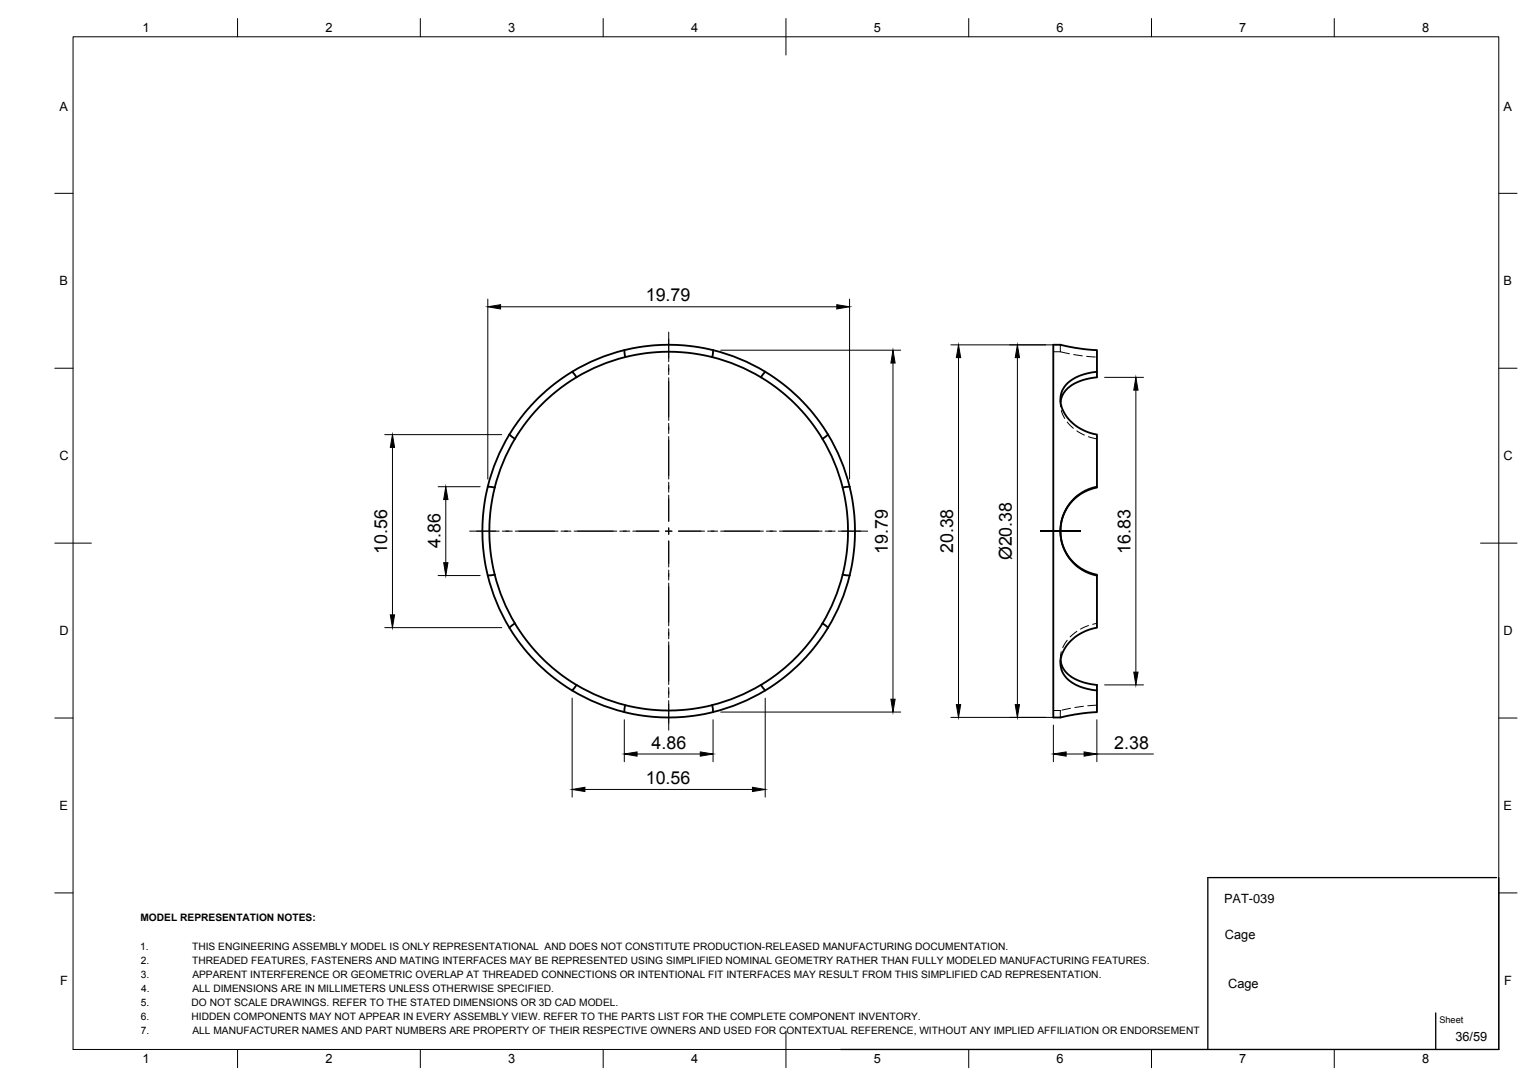
ISO-10303-21;
HEADER;
/* Generated by software containing ST-Developer
 * from STEP Tools, Inc. (www.steptools.com) 
 */

FILE_DESCRIPTION(
/* description */ ('Four-bar parallelogram arm'),
/* implementation_level */ '2;1');

FILE_NAME(
/* name */ 'Cage.step',
/* time_stamp */ '2026-10-28T03:24:55-07:00',
/* author */ (''),
/* organization */ (''),
/* preprocessor_version */ 'ST-DEVELOPER v20.2',
/* originating_system */ 'Autodesk Translation Framework v15.17.0.0',
/* authorisation */ '');

FILE_SCHEMA (('AUTOMOTIVE_DESIGN { 1 0 10303 214 3 1 1 }'));
ENDSEC;

DATA;
#10=MECHANICAL_DESIGN_GEOMETRIC_PRESENTATION_REPRESENTATION('',(#664),#14512);
#467=SPHERICAL_SURFACE('',#8565,0.247676);
#468=SPHERICAL_SURFACE('',#8581,0.247676);
#469=SPHERICAL_SURFACE('',#8586,0.247676);
#470=SPHERICAL_SURFACE('',#8591,0.247676);
#471=SPHERICAL_SURFACE('',#8596,0.247676);
#472=SPHERICAL_SURFACE('',#8601,0.247676);
#473=SPHERICAL_SURFACE('',#8606,0.247676);
#474=SPHERICAL_SURFACE('',#8614,0.247676);
#504=B_SPLINE_CURVE_WITH_KNOTS('',3,(#13344,#13345,#13346,#13347,#13348,
#13349,#13350,#13351,#13352,#13353,#13354,#13355,#13356,#13357,#13358,#13359,
#13360,#13361,#13362,#13363,#13364,#13365),.UNSPECIFIED.,.F.,.F.,(4,2,2,
2,2,2,2,2,2,2,4),(0.0473477652366656,0.126350602536658,0.189525903804987,
0.252701205073317,0.313298422430275,0.373895639787233,0.434492857144191,
0.495090074501149,0.558265375769478,0.621440677037807,0.7004435143378),
 .UNSPECIFIED.);
#505=B_SPLINE_CURVE_WITH_KNOTS('',3,(#13369,#13370,#13371,#13372,#13373,
#13374,#13375,#13376,#13377,#13378,#13379,#13380,#13381,#13382,#13383,#13384,
#13385,#13386,#13387,#13388,#13389,#13390),.UNSPECIFIED.,.F.,.F.,(4,2,2,
2,2,2,2,2,2,2,4),(0.0464897534940957,0.0852567806515119,0.170513561303024,
0.246687263103517,0.308657850341199,0.370628437578881,0.432599024816563,
0.494569612054245,0.570743313854739,0.656000094506251,0.694767121663666),
 .UNSPECIFIED.);
#506=B_SPLINE_CURVE_WITH_KNOTS('',3,(#13396,#13397,#13398,#13399,#13400,
#13401,#13402,#13403,#13404,#13405,#13406,#13407,#13408,#13409,#13410,#13411,
#13412,#13413,#13414,#13415,#13416,#13417),.UNSPECIFIED.,.F.,.F.,(4,2,2,
2,2,2,2,2,2,2,4),(0.0464897534940957,0.0852567806515118,0.170513561303024,
0.246687263103517,0.308657850341199,0.370628437578881,0.432599024816563,
0.494569612054245,0.570743313854738,0.65600009450625,0.694767121663666),
 .UNSPECIFIED.);
#507=B_SPLINE_CURVE_WITH_KNOTS('',3,(#13421,#13422,#13423,#13424,#13425,
#13426,#13427,#13428,#13429,#13430,#13431,#13432,#13433,#13434,#13435,#13436,
#13437,#13438,#13439,#13440,#13441,#13442),.UNSPECIFIED.,.F.,.F.,(4,2,2,
2,2,2,2,2,2,2,4),(0.0464897534940957,0.0852567806515119,0.170513561303024,
0.246687263103517,0.308657850341199,0.370628437578881,0.432599024816563,
0.494569612054245,0.570743313854739,0.656000094506251,0.694767121663666),
 .UNSPECIFIED.);
#508=B_SPLINE_CURVE_WITH_KNOTS('',3,(#13446,#13447,#13448,#13449,#13450,
#13451,#13452,#13453,#13454,#13455,#13456,#13457),.UNSPECIFIED.,.F.,.F.,
(4,2,2,2,2,4),(0.0464897534940957,0.0852567806515119,0.170513561303024,
0.246687263103517,0.308657850341199,0.370628437578881),.UNSPECIFIED.);
#509=B_SPLINE_CURVE_WITH_KNOTS('',3,(#13462,#13463,#13464,#13465,#13466,
#13467,#13468,#13469,#13470,#13471,#13472,#13473),.UNSPECIFIED.,.F.,.F.,
(4,2,2,2,2,4),(0.370628437578881,0.432599024816563,0.494569612054245,0.570743313854738,
0.65600009450625,0.694767121663666),.UNSPECIFIED.);
#510=B_SPLINE_CURVE_WITH_KNOTS('',3,(#13477,#13478,#13479,#13480,#13481,
#13482,#13483,#13484,#13485,#13486,#13487,#13488,#13489,#13490,#13491,#13492,
#13493,#13494,#13495,#13496,#13497,#13498),.UNSPECIFIED.,.F.,.F.,(4,2,2,
2,2,2,2,2,2,2,4),(0.0464897534940957,0.0852567806515121,0.170513561303024,
0.246687263103518,0.308657850341199,0.370628437578881,0.432599024816563,
0.494569612054245,0.570743313854738,0.65600009450625,0.694767121663666),
 .UNSPECIFIED.);
#511=B_SPLINE_CURVE_WITH_KNOTS('',3,(#13502,#13503,#13504,#13505,#13506,
#13507,#13508,#13509,#13510,#13511,#13512,#13513,#13514,#13515,#13516,#13517,
#13518,#13519,#13520,#13521,#13522,#13523),.UNSPECIFIED.,.F.,.F.,(4,2,2,
2,2,2,2,2,2,2,4),(0.0464897534940957,0.0852567806515119,0.170513561303024,
0.246687263103517,0.308657850341199,0.370628437578881,0.432599024816563,
0.494569612054245,0.570743313854738,0.65600009450625,0.694767121663667),
 .UNSPECIFIED.);
#512=B_SPLINE_CURVE_WITH_KNOTS('',3,(#13527,#13528,#13529,#13530,#13531,
#13532,#13533,#13534,#13535,#13536,#13537,#13538,#13539,#13540,#13541,#13542,
#13543,#13544,#13545,#13546,#13547,#13548),.UNSPECIFIED.,.F.,.F.,(4,2,2,
2,2,2,2,2,2,2,4),(0.0464897534940957,0.0852567806515119,0.170513561303024,
0.246687263103517,0.308657850341199,0.370628437578881,0.432599024816563,
0.494569612054245,0.570743313854738,0.65600009450625,0.694767121663666),
 .UNSPECIFIED.);
#513=B_SPLINE_CURVE_WITH_KNOTS('',3,(#13552,#13553,#13554,#13555,#13556,
#13557,#13558,#13559,#13560,#13561,#13562,#13563,#13564,#13565,#13566,#13567,
#13568,#13569,#13570,#13571,#13572,#13573),.UNSPECIFIED.,.F.,.F.,(4,2,2,
2,2,2,2,2,2,2,4),(0.0464897534940957,0.0852567806515119,0.170513561303024,
0.246687263103517,0.308657850341199,0.370628437578881,0.432599024816563,
0.494569612054245,0.570743313854739,0.656000094506251,0.694767121663667),
 .UNSPECIFIED.);
#514=B_SPLINE_CURVE_WITH_KNOTS('',3,(#13581,#13582,#13583,#13584,#13585,
#13586,#13587,#13588,#13589,#13590,#13591,#13592,#13593,#13594,#13595,#13596,
#13597,#13598,#13599,#13600,#13601,#13602),.UNSPECIFIED.,.F.,.F.,(4,2,2,
2,2,2,2,2,2,2,4),(0.0473477652366656,0.126350602536658,0.189525903804987,
0.252701205073316,0.313298422430274,0.373895639787232,0.434492857144191,
0.495090074501149,0.558265375769478,0.621440677037807,0.7004435143378),
 .UNSPECIFIED.);
#515=B_SPLINE_CURVE_WITH_KNOTS('',3,(#13610,#13611,#13612,#13613,#13614,
#13615,#13616,#13617,#13618,#13619,#13620,#13621,#13622,#13623,#13624,#13625,
#13626,#13627,#13628,#13629,#13630,#13631),.UNSPECIFIED.,.F.,.F.,(4,2,2,
2,2,2,2,2,2,2,4),(0.0473477652366656,0.126350602536658,0.189525903804987,
0.252701205073317,0.313298422430275,0.373895639787233,0.434492857144191,
0.495090074501149,0.558265375769478,0.621440677037807,0.7004435143378),
 .UNSPECIFIED.);
#516=B_SPLINE_CURVE_WITH_KNOTS('',3,(#13640,#13641,#13642,#13643,#13644,
#13645,#13646,#13647,#13648,#13649,#13650,#13651),.UNSPECIFIED.,.F.,.F.,
(4,2,2,2,2,4),(0.0473477652366656,0.126350602536658,0.189525903804987,0.252701205073316,
0.313298422430275,0.373895639787233),.UNSPECIFIED.);
#517=B_SPLINE_CURVE_WITH_KNOTS('',3,(#13653,#13654,#13655,#13656,#13657,
#13658,#13659,#13660,#13661,#13662,#13663,#13664),.UNSPECIFIED.,.F.,.F.,
(4,2,2,2,2,4),(0.373895639787233,0.434492857144191,0.495090074501149,0.558265375769478,
0.621440677037807,0.7004435143378),.UNSPECIFIED.);
#518=B_SPLINE_CURVE_WITH_KNOTS('',3,(#13671,#13672,#13673,#13674,#13675,
#13676,#13677,#13678,#13679,#13680,#13681,#13682,#13683,#13684,#13685,#13686,
#13687,#13688,#13689,#13690,#13691,#13692),.UNSPECIFIED.,.F.,.F.,(4,2,2,
2,2,2,2,2,2,2,4),(0.0473477652366656,0.126350602536658,0.189525903804987,
0.252701205073316,0.313298422430275,0.373895639787233,0.434492857144191,
0.495090074501149,0.558265375769478,0.621440677037807,0.7004435143378),
 .UNSPECIFIED.);
#519=B_SPLINE_CURVE_WITH_KNOTS('',3,(#13700,#13701,#13702,#13703,#13704,
#13705,#13706,#13707,#13708,#13709,#13710,#13711,#13712,#13713,#13714,#13715,
#13716,#13717,#13718,#13719,#13720,#13721),.UNSPECIFIED.,.F.,.F.,(4,2,2,
2,2,2,2,2,2,2,4),(0.0473477652366656,0.126350602536658,0.189525903804987,
0.252701205073317,0.313298422430275,0.373895639787233,0.434492857144191,
0.495090074501149,0.558265375769478,0.621440677037807,0.7004435143378),
 .UNSPECIFIED.);
#520=B_SPLINE_CURVE_WITH_KNOTS('',3,(#13729,#13730,#13731,#13732,#13733,
#13734,#13735,#13736,#13737,#13738,#13739,#13740,#13741,#13742,#13743,#13744,
#13745,#13746,#13747,#13748,#13749,#13750),.UNSPECIFIED.,.F.,.F.,(4,2,2,
2,2,2,2,2,2,2,4),(0.0473477652366656,0.126350602536658,0.189525903804987,
0.252701205073316,0.313298422430275,0.373895639787233,0.434492857144191,
0.495090074501149,0.558265375769478,0.621440677037807,0.7004435143378),
 .UNSPECIFIED.);
#521=B_SPLINE_CURVE_WITH_KNOTS('',3,(#13759,#13760,#13761,#13762,#13763,
#13764,#13765,#13766,#13767,#13768,#13769,#13770,#13771,#13772,#13773,#13774,
#13775,#13776,#13777,#13778,#13779,#13780),.UNSPECIFIED.,.F.,.F.,(4,2,2,
2,2,2,2,2,2,2,4),(0.0473477652366656,0.126350602536658,0.189525903804987,
0.252701205073317,0.313298422430275,0.373895639787233,0.434492857144191,
0.495090074501149,0.558265375769478,0.621440677037807,0.7004435143378),
 .UNSPECIFIED.);
#557=SHAPE_REPRESENTATION_RELATIONSHIP('SRR','None',#14781,#607);
#607=ADVANCED_BREP_SHAPE_REPRESENTATION('',(#721),#14496);
#664=STYLED_ITEM('',(#15087),#721);
#721=MANIFOLD_SOLID_BREP('Continuous crown cage',#7369);
#941=FACE_BOUND('',#2128,.T.);
#1131=PLANE('',#8578);
#1132=PLANE('',#8583);
#1133=PLANE('',#8588);
#1134=PLANE('',#8593);
#1135=PLANE('',#8598);
#1136=PLANE('',#8603);
#1137=PLANE('',#8612);
#1138=PLANE('',#8616);
#1139=PLANE('',#8617);
#1484=FACE_OUTER_BOUND('',#2110,.T.);
#1485=FACE_OUTER_BOUND('',#2111,.T.);
#1486=FACE_OUTER_BOUND('',#2112,.T.);
#1487=FACE_OUTER_BOUND('',#2113,.T.);
#1488=FACE_OUTER_BOUND('',#2114,.T.);
#1489=FACE_OUTER_BOUND('',#2115,.T.);
#1490=FACE_OUTER_BOUND('',#2116,.T.);
#1491=FACE_OUTER_BOUND('',#2117,.T.);
#1492=FACE_OUTER_BOUND('',#2118,.T.);
#1493=FACE_OUTER_BOUND('',#2119,.T.);
#1494=FACE_OUTER_BOUND('',#2120,.T.);
#1495=FACE_OUTER_BOUND('',#2121,.T.);
#1496=FACE_OUTER_BOUND('',#2122,.T.);
#1497=FACE_OUTER_BOUND('',#2123,.T.);
#1498=FACE_OUTER_BOUND('',#2124,.T.);
#1499=FACE_OUTER_BOUND('',#2125,.T.);
#1500=FACE_OUTER_BOUND('',#2126,.T.);
#1501=FACE_OUTER_BOUND('',#2127,.T.);
#1502=FACE_OUTER_BOUND('',#2129,.T.);
#2110=EDGE_LOOP('',(#6164,#6165,#6166,#6167));
#2111=EDGE_LOOP('',(#6168,#6169,#6170,#6171,#6172,#6173,#6174,#6175,#6176,
#6177,#6178,#6179,#6180,#6181,#6182,#6183,#6184,#6185,#6186,#6187));
#2112=EDGE_LOOP('',(#6188,#6189,#6190,#6191));
#2113=EDGE_LOOP('',(#6192,#6193,#6194,#6195));
#2114=EDGE_LOOP('',(#6196,#6197,#6198,#6199));
#2115=EDGE_LOOP('',(#6200,#6201,#6202,#6203));
#2116=EDGE_LOOP('',(#6204,#6205,#6206,#6207));
#2117=EDGE_LOOP('',(#6208,#6209,#6210,#6211,#6212,#6213));
#2118=EDGE_LOOP('',(#6214,#6215,#6216,#6217));
#2119=EDGE_LOOP('',(#6218,#6219,#6220,#6221));
#2120=EDGE_LOOP('',(#6222,#6223,#6224,#6225));
#2121=EDGE_LOOP('',(#6226,#6227,#6228,#6229));
#2122=EDGE_LOOP('',(#6230,#6231,#6232,#6233));
#2123=EDGE_LOOP('',(#6234,#6235,#6236,#6237));
#2124=EDGE_LOOP('',(#6238,#6239,#6240,#6241,#6242,#6243,#6244,#6245,#6246,
#6247,#6248,#6249,#6250,#6251,#6252,#6253,#6254,#6255,#6256,#6257));
#2125=EDGE_LOOP('',(#6258,#6259,#6260,#6261));
#2126=EDGE_LOOP('',(#6262,#6263,#6264,#6265));
#2127=EDGE_LOOP('',(#6266));
#2128=EDGE_LOOP('',(#6267));
#2129=EDGE_LOOP('',(#6268,#6269,#6270,#6271));
#2590=LINE('',#13459,#2984);
#2591=LINE('',#13755,#2985);
#2984=VECTOR('',#10516,1.019052);
#2985=VECTOR('',#10593,0.980948);
#3404=CIRCLE('',#8566,0.243053047864041);
#3405=CIRCLE('',#8567,0.243053047864041);
#3406=CIRCLE('',#8569,1.019052);
#3407=CIRCLE('',#8570,1.019052);
#3408=CIRCLE('',#8571,1.019052);
#3409=CIRCLE('',#8572,1.019052);
#3410=CIRCLE('',#8573,1.019052);
#3411=CIRCLE('',#8574,1.019052);
#3412=CIRCLE('',#8575,1.019052);
#3413=CIRCLE('',#8576,1.019052);
#3414=CIRCLE('',#8577,1.019052);
#3415=CIRCLE('',#8579,0.980948);
#3416=CIRCLE('',#8580,0.243053047864041);
#3417=CIRCLE('',#8582,0.243053047864041);
#3418=CIRCLE('',#8584,0.980948);
#3419=CIRCLE('',#8585,0.243053047864041);
#3420=CIRCLE('',#8587,0.243053047864041);
#3421=CIRCLE('',#8589,0.980948);
#3422=CIRCLE('',#8590,0.243053047864041);
#3423=CIRCLE('',#8592,0.243053047864041);
#3424=CIRCLE('',#8594,0.980948);
#3425=CIRCLE('',#8595,0.243053047864041);
#3426=CIRCLE('',#8597,0.243053047864041);
#3427=CIRCLE('',#8599,0.980948);
#3428=CIRCLE('',#8600,0.243053047864041);
#3429=CIRCLE('',#8602,0.243053047864041);
#3430=CIRCLE('',#8604,0.980948);
#3431=CIRCLE('',#8605,0.243053047864041);
#3432=CIRCLE('',#8607,0.243053047864041);
#3433=CIRCLE('',#8609,0.980948);
#3434=CIRCLE('',#8610,0.980948);
#3435=CIRCLE('',#8611,0.980948);
#3436=CIRCLE('',#8613,0.243053047864041);
#3437=CIRCLE('',#8615,0.243053047864041);
#3944=VERTEX_POINT('',#13342);
#3945=VERTEX_POINT('',#13343);
#3946=VERTEX_POINT('',#13366);
#3947=VERTEX_POINT('',#13368);
#3948=VERTEX_POINT('',#13393);
#3949=VERTEX_POINT('',#13395);
#3950=VERTEX_POINT('',#13418);
#3951=VERTEX_POINT('',#13420);
#3952=VERTEX_POINT('',#13443);
#3953=VERTEX_POINT('',#13445);
#3954=VERTEX_POINT('',#13458);
#3955=VERTEX_POINT('',#13461);
#3956=VERTEX_POINT('',#13474);
#3957=VERTEX_POINT('',#13476);
#3958=VERTEX_POINT('',#13499);
#3959=VERTEX_POINT('',#13501);
#3960=VERTEX_POINT('',#13524);
#3961=VERTEX_POINT('',#13526);
#3962=VERTEX_POINT('',#13549);
#3963=VERTEX_POINT('',#13551);
#3964=VERTEX_POINT('',#13576);
#3965=VERTEX_POINT('',#13580);
#3966=VERTEX_POINT('',#13605);
#3967=VERTEX_POINT('',#13609);
#3968=VERTEX_POINT('',#13634);
#3969=VERTEX_POINT('',#13638);
#3970=VERTEX_POINT('',#13639);
#3971=VERTEX_POINT('',#13666);
#3972=VERTEX_POINT('',#13670);
#3973=VERTEX_POINT('',#13695);
#3974=VERTEX_POINT('',#13699);
#3975=VERTEX_POINT('',#13724);
#3976=VERTEX_POINT('',#13728);
#3977=VERTEX_POINT('',#13753);
#3978=VERTEX_POINT('',#13756);
#3979=VERTEX_POINT('',#13758);
#4713=EDGE_CURVE('',#3944,#3945,#504,.T.);
#4714=EDGE_CURVE('',#3946,#3944,#3404,.T.);
#4715=EDGE_CURVE('',#3947,#3946,#505,.T.);
#4716=EDGE_CURVE('',#3945,#3947,#3405,.T.);
#4717=EDGE_CURVE('',#3948,#3946,#3406,.T.);
#4718=EDGE_CURVE('',#3948,#3949,#506,.T.);
#4719=EDGE_CURVE('',#3950,#3949,#3407,.T.);
#4720=EDGE_CURVE('',#3950,#3951,#507,.T.);
#4721=EDGE_CURVE('',#3952,#3951,#3408,.T.);
#4722=EDGE_CURVE('',#3952,#3953,#508,.T.);
#4723=EDGE_CURVE('',#3953,#3954,#2590,.T.);
#4724=EDGE_CURVE('',#3954,#3954,#3409,.T.);
#4725=EDGE_CURVE('',#3953,#3955,#509,.T.);
#4726=EDGE_CURVE('',#3956,#3955,#3410,.T.);
#4727=EDGE_CURVE('',#3956,#3957,#510,.T.);
#4728=EDGE_CURVE('',#3958,#3957,#3411,.T.);
#4729=EDGE_CURVE('',#3958,#3959,#511,.T.);
#4730=EDGE_CURVE('',#3960,#3959,#3412,.T.);
#4731=EDGE_CURVE('',#3960,#3961,#512,.T.);
#4732=EDGE_CURVE('',#3962,#3961,#3413,.T.);
#4733=EDGE_CURVE('',#3962,#3963,#513,.T.);
#4734=EDGE_CURVE('',#3947,#3963,#3414,.T.);
#4735=EDGE_CURVE('',#3944,#3964,#3415,.T.);
#4736=EDGE_CURVE('',#3964,#3948,#3416,.T.);
#4737=EDGE_CURVE('',#3965,#3964,#514,.T.);
#4738=EDGE_CURVE('',#3949,#3965,#3417,.T.);
#4739=EDGE_CURVE('',#3965,#3966,#3418,.T.);
#4740=EDGE_CURVE('',#3966,#3950,#3419,.T.);
#4741=EDGE_CURVE('',#3967,#3966,#515,.T.);
#4742=EDGE_CURVE('',#3951,#3967,#3420,.T.);
#4743=EDGE_CURVE('',#3967,#3968,#3421,.T.);
#4744=EDGE_CURVE('',#3968,#3952,#3422,.T.);
#4745=EDGE_CURVE('',#3969,#3970,#516,.T.);
#4746=EDGE_CURVE('',#3955,#3969,#3423,.T.);
#4747=EDGE_CURVE('',#3970,#3968,#517,.T.);
#4748=EDGE_CURVE('',#3969,#3971,#3424,.T.);
#4749=EDGE_CURVE('',#3971,#3956,#3425,.T.);
#4750=EDGE_CURVE('',#3972,#3971,#518,.T.);
#4751=EDGE_CURVE('',#3957,#3972,#3426,.T.);
#4752=EDGE_CURVE('',#3972,#3973,#3427,.T.);
#4753=EDGE_CURVE('',#3973,#3958,#3428,.T.);
#4754=EDGE_CURVE('',#3974,#3973,#519,.T.);
#4755=EDGE_CURVE('',#3959,#3974,#3429,.T.);
#4756=EDGE_CURVE('',#3974,#3975,#3430,.T.);
#4757=EDGE_CURVE('',#3975,#3960,#3431,.T.);
#4758=EDGE_CURVE('',#3976,#3975,#520,.T.);
#4759=EDGE_CURVE('',#3961,#3976,#3432,.T.);
#4760=EDGE_CURVE('',#3977,#3977,#3433,.T.);
#4761=EDGE_CURVE('',#3977,#3970,#2591,.T.);
#4762=EDGE_CURVE('',#3978,#3945,#3434,.T.);
#4763=EDGE_CURVE('',#3978,#3979,#521,.T.);
#4764=EDGE_CURVE('',#3976,#3979,#3435,.T.);
#4765=EDGE_CURVE('',#3963,#3978,#3436,.T.);
#4766=EDGE_CURVE('',#3979,#3962,#3437,.T.);
#6164=ORIENTED_EDGE('',*,*,#4713,.F.);
#6165=ORIENTED_EDGE('',*,*,#4714,.F.);
#6166=ORIENTED_EDGE('',*,*,#4715,.F.);
#6167=ORIENTED_EDGE('',*,*,#4716,.F.);
#6168=ORIENTED_EDGE('',*,*,#4715,.T.);
#6169=ORIENTED_EDGE('',*,*,#4717,.F.);
#6170=ORIENTED_EDGE('',*,*,#4718,.T.);
#6171=ORIENTED_EDGE('',*,*,#4719,.F.);
#6172=ORIENTED_EDGE('',*,*,#4720,.T.);
#6173=ORIENTED_EDGE('',*,*,#4721,.F.);
#6174=ORIENTED_EDGE('',*,*,#4722,.T.);
#6175=ORIENTED_EDGE('',*,*,#4723,.T.);
#6176=ORIENTED_EDGE('',*,*,#4724,.F.);
#6177=ORIENTED_EDGE('',*,*,#4723,.F.);
#6178=ORIENTED_EDGE('',*,*,#4725,.T.);
#6179=ORIENTED_EDGE('',*,*,#4726,.F.);
#6180=ORIENTED_EDGE('',*,*,#4727,.T.);
#6181=ORIENTED_EDGE('',*,*,#4728,.F.);
#6182=ORIENTED_EDGE('',*,*,#4729,.T.);
#6183=ORIENTED_EDGE('',*,*,#4730,.F.);
#6184=ORIENTED_EDGE('',*,*,#4731,.T.);
#6185=ORIENTED_EDGE('',*,*,#4732,.F.);
#6186=ORIENTED_EDGE('',*,*,#4733,.T.);
#6187=ORIENTED_EDGE('',*,*,#4734,.F.);
#6188=ORIENTED_EDGE('',*,*,#4714,.T.);
#6189=ORIENTED_EDGE('',*,*,#4735,.T.);
#6190=ORIENTED_EDGE('',*,*,#4736,.T.);
#6191=ORIENTED_EDGE('',*,*,#4717,.T.);
#6192=ORIENTED_EDGE('',*,*,#4737,.F.);
#6193=ORIENTED_EDGE('',*,*,#4738,.F.);
#6194=ORIENTED_EDGE('',*,*,#4718,.F.);
#6195=ORIENTED_EDGE('',*,*,#4736,.F.);
#6196=ORIENTED_EDGE('',*,*,#4738,.T.);
#6197=ORIENTED_EDGE('',*,*,#4739,.T.);
#6198=ORIENTED_EDGE('',*,*,#4740,.T.);
#6199=ORIENTED_EDGE('',*,*,#4719,.T.);
#6200=ORIENTED_EDGE('',*,*,#4741,.F.);
#6201=ORIENTED_EDGE('',*,*,#4742,.F.);
#6202=ORIENTED_EDGE('',*,*,#4720,.F.);
#6203=ORIENTED_EDGE('',*,*,#4740,.F.);
#6204=ORIENTED_EDGE('',*,*,#4742,.T.);
#6205=ORIENTED_EDGE('',*,*,#4743,.T.);
#6206=ORIENTED_EDGE('',*,*,#4744,.T.);
#6207=ORIENTED_EDGE('',*,*,#4721,.T.);
#6208=ORIENTED_EDGE('',*,*,#4745,.F.);
#6209=ORIENTED_EDGE('',*,*,#4746,.F.);
#6210=ORIENTED_EDGE('',*,*,#4725,.F.);
#6211=ORIENTED_EDGE('',*,*,#4722,.F.);
#6212=ORIENTED_EDGE('',*,*,#4744,.F.);
#6213=ORIENTED_EDGE('',*,*,#4747,.F.);
#6214=ORIENTED_EDGE('',*,*,#4746,.T.);
#6215=ORIENTED_EDGE('',*,*,#4748,.T.);
#6216=ORIENTED_EDGE('',*,*,#4749,.T.);
#6217=ORIENTED_EDGE('',*,*,#4726,.T.);
#6218=ORIENTED_EDGE('',*,*,#4750,.F.);
#6219=ORIENTED_EDGE('',*,*,#4751,.F.);
#6220=ORIENTED_EDGE('',*,*,#4727,.F.);
#6221=ORIENTED_EDGE('',*,*,#4749,.F.);
#6222=ORIENTED_EDGE('',*,*,#4751,.T.);
#6223=ORIENTED_EDGE('',*,*,#4752,.T.);
#6224=ORIENTED_EDGE('',*,*,#4753,.T.);
#6225=ORIENTED_EDGE('',*,*,#4728,.T.);
#6226=ORIENTED_EDGE('',*,*,#4754,.F.);
#6227=ORIENTED_EDGE('',*,*,#4755,.F.);
#6228=ORIENTED_EDGE('',*,*,#4729,.F.);
#6229=ORIENTED_EDGE('',*,*,#4753,.F.);
#6230=ORIENTED_EDGE('',*,*,#4755,.T.);
#6231=ORIENTED_EDGE('',*,*,#4756,.T.);
#6232=ORIENTED_EDGE('',*,*,#4757,.T.);
#6233=ORIENTED_EDGE('',*,*,#4730,.T.);
#6234=ORIENTED_EDGE('',*,*,#4731,.F.);
#6235=ORIENTED_EDGE('',*,*,#4757,.F.);
#6236=ORIENTED_EDGE('',*,*,#4758,.F.);
#6237=ORIENTED_EDGE('',*,*,#4759,.F.);
#6238=ORIENTED_EDGE('',*,*,#4760,.F.);
#6239=ORIENTED_EDGE('',*,*,#4761,.T.);
#6240=ORIENTED_EDGE('',*,*,#4747,.T.);
#6241=ORIENTED_EDGE('',*,*,#4743,.F.);
#6242=ORIENTED_EDGE('',*,*,#4741,.T.);
#6243=ORIENTED_EDGE('',*,*,#4739,.F.);
#6244=ORIENTED_EDGE('',*,*,#4737,.T.);
#6245=ORIENTED_EDGE('',*,*,#4735,.F.);
#6246=ORIENTED_EDGE('',*,*,#4713,.T.);
#6247=ORIENTED_EDGE('',*,*,#4762,.F.);
#6248=ORIENTED_EDGE('',*,*,#4763,.T.);
#6249=ORIENTED_EDGE('',*,*,#4764,.F.);
#6250=ORIENTED_EDGE('',*,*,#4758,.T.);
#6251=ORIENTED_EDGE('',*,*,#4756,.F.);
#6252=ORIENTED_EDGE('',*,*,#4754,.T.);
#6253=ORIENTED_EDGE('',*,*,#4752,.F.);
#6254=ORIENTED_EDGE('',*,*,#4750,.T.);
#6255=ORIENTED_EDGE('',*,*,#4748,.F.);
#6256=ORIENTED_EDGE('',*,*,#4745,.T.);
#6257=ORIENTED_EDGE('',*,*,#4761,.F.);
#6258=ORIENTED_EDGE('',*,*,#4716,.T.);
#6259=ORIENTED_EDGE('',*,*,#4734,.T.);
#6260=ORIENTED_EDGE('',*,*,#4765,.T.);
#6261=ORIENTED_EDGE('',*,*,#4762,.T.);
#6262=ORIENTED_EDGE('',*,*,#4733,.F.);
#6263=ORIENTED_EDGE('',*,*,#4766,.F.);
#6264=ORIENTED_EDGE('',*,*,#4763,.F.);
#6265=ORIENTED_EDGE('',*,*,#4765,.F.);
#6266=ORIENTED_EDGE('',*,*,#4724,.T.);
#6267=ORIENTED_EDGE('',*,*,#4760,.T.);
#6268=ORIENTED_EDGE('',*,*,#4759,.T.);
#6269=ORIENTED_EDGE('',*,*,#4764,.T.);
#6270=ORIENTED_EDGE('',*,*,#4766,.T.);
#6271=ORIENTED_EDGE('',*,*,#4732,.T.);
#6854=CYLINDRICAL_SURFACE('',#8568,1.019052);
#6855=CYLINDRICAL_SURFACE('',#8608,0.980948);
#7189=ADVANCED_FACE('',(#1484),#467,.F.);
#7190=ADVANCED_FACE('',(#1485),#6854,.T.);
#7191=ADVANCED_FACE('',(#1486),#1131,.T.);
#7192=ADVANCED_FACE('',(#1487),#468,.F.);
#7193=ADVANCED_FACE('',(#1488),#1132,.T.);
#7194=ADVANCED_FACE('',(#1489),#469,.F.);
#7195=ADVANCED_FACE('',(#1490),#1133,.T.);
#7196=ADVANCED_FACE('',(#1491),#470,.F.);
#7197=ADVANCED_FACE('',(#1492),#1134,.T.);
#7198=ADVANCED_FACE('',(#1493),#471,.F.);
#7199=ADVANCED_FACE('',(#1494),#1135,.T.);
#7200=ADVANCED_FACE('',(#1495),#472,.F.);
#7201=ADVANCED_FACE('',(#1496),#1136,.T.);
#7202=ADVANCED_FACE('',(#1497),#473,.F.);
#7203=ADVANCED_FACE('',(#1498),#6855,.F.);
#7204=ADVANCED_FACE('',(#1499),#1137,.T.);
#7205=ADVANCED_FACE('',(#1500),#474,.F.);
#7206=ADVANCED_FACE('',(#1501,#941),#1138,.T.);
#7207=ADVANCED_FACE('',(#1502),#1139,.T.);
#7369=CLOSED_SHELL('',(#7189,#7190,#7191,#7192,#7193,#7194,#7195,#7196,
#7197,#7198,#7199,#7200,#7201,#7202,#7203,#7204,#7205,#7206,#7207));
#8564=AXIS2_PLACEMENT_3D('',#13340,#10500,#10501);
#8565=AXIS2_PLACEMENT_3D('',#13341,#10502,#10503);
#8566=AXIS2_PLACEMENT_3D('',#13367,#10504,#10505);
#8567=AXIS2_PLACEMENT_3D('',#13391,#10506,#10507);
#8568=AXIS2_PLACEMENT_3D('',#13392,#10508,#10509);
#8569=AXIS2_PLACEMENT_3D('',#13394,#10510,#10511);
#8570=AXIS2_PLACEMENT_3D('',#13419,#10512,#10513);
#8571=AXIS2_PLACEMENT_3D('',#13444,#10514,#10515);
#8572=AXIS2_PLACEMENT_3D('',#13460,#10517,#10518);
#8573=AXIS2_PLACEMENT_3D('',#13475,#10519,#10520);
#8574=AXIS2_PLACEMENT_3D('',#13500,#10521,#10522);
#8575=AXIS2_PLACEMENT_3D('',#13525,#10523,#10524);
#8576=AXIS2_PLACEMENT_3D('',#13550,#10525,#10526);
#8577=AXIS2_PLACEMENT_3D('',#13574,#10527,#10528);
#8578=AXIS2_PLACEMENT_3D('',#13575,#10529,#10530);
#8579=AXIS2_PLACEMENT_3D('',#13577,#10531,#10532);
#8580=AXIS2_PLACEMENT_3D('',#13578,#10533,#10534);
#8581=AXIS2_PLACEMENT_3D('',#13579,#10535,#10536);
#8582=AXIS2_PLACEMENT_3D('',#13603,#10537,#10538);
#8583=AXIS2_PLACEMENT_3D('',#13604,#10539,#10540);
#8584=AXIS2_PLACEMENT_3D('',#13606,#10541,#10542);
#8585=AXIS2_PLACEMENT_3D('',#13607,#10543,#10544);
#8586=AXIS2_PLACEMENT_3D('',#13608,#10545,#10546);
#8587=AXIS2_PLACEMENT_3D('',#13632,#10547,#10548);
#8588=AXIS2_PLACEMENT_3D('',#13633,#10549,#10550);
#8589=AXIS2_PLACEMENT_3D('',#13635,#10551,#10552);
#8590=AXIS2_PLACEMENT_3D('',#13636,#10553,#10554);
#8591=AXIS2_PLACEMENT_3D('',#13637,#10555,#10556);
#8592=AXIS2_PLACEMENT_3D('',#13652,#10557,#10558);
#8593=AXIS2_PLACEMENT_3D('',#13665,#10559,#10560);
#8594=AXIS2_PLACEMENT_3D('',#13667,#10561,#10562);
#8595=AXIS2_PLACEMENT_3D('',#13668,#10563,#10564);
#8596=AXIS2_PLACEMENT_3D('',#13669,#10565,#10566);
#8597=AXIS2_PLACEMENT_3D('',#13693,#10567,#10568);
#8598=AXIS2_PLACEMENT_3D('',#13694,#10569,#10570);
#8599=AXIS2_PLACEMENT_3D('',#13696,#10571,#10572);
#8600=AXIS2_PLACEMENT_3D('',#13697,#10573,#10574);
#8601=AXIS2_PLACEMENT_3D('',#13698,#10575,#10576);
#8602=AXIS2_PLACEMENT_3D('',#13722,#10577,#10578);
#8603=AXIS2_PLACEMENT_3D('',#13723,#10579,#10580);
#8604=AXIS2_PLACEMENT_3D('',#13725,#10581,#10582);
#8605=AXIS2_PLACEMENT_3D('',#13726,#10583,#10584);
#8606=AXIS2_PLACEMENT_3D('',#13727,#10585,#10586);
#8607=AXIS2_PLACEMENT_3D('',#13751,#10587,#10588);
#8608=AXIS2_PLACEMENT_3D('',#13752,#10589,#10590);
#8609=AXIS2_PLACEMENT_3D('',#13754,#10591,#10592);
#8610=AXIS2_PLACEMENT_3D('',#13757,#10594,#10595);
#8611=AXIS2_PLACEMENT_3D('',#13781,#10596,#10597);
#8612=AXIS2_PLACEMENT_3D('',#13782,#10598,#10599);
#8613=AXIS2_PLACEMENT_3D('',#13783,#10600,#10601);
#8614=AXIS2_PLACEMENT_3D('',#13784,#10602,#10603);
#8615=AXIS2_PLACEMENT_3D('',#13785,#10604,#10605);
#8616=AXIS2_PLACEMENT_3D('',#13786,#10606,#10607);
#8617=AXIS2_PLACEMENT_3D('',#13787,#10608,#10609);
#10500=DIRECTION('axis',(0.,0.,1.));
#10501=DIRECTION('refdir',(1.,0.,0.));
#10502=DIRECTION('center_axis',(0.,0.,1.));
#10503=DIRECTION('ref_axis',(1.,0.,0.));
#10504=DIRECTION('center_axis',(0.,-1.,0.));
#10505=DIRECTION('ref_axis',(0.,0.,-1.));
#10506=DIRECTION('center_axis',(0.,-1.,0.));
#10507=DIRECTION('ref_axis',(0.,0.,-1.));
#10508=DIRECTION('center_axis',(0.,1.,0.));
#10509=DIRECTION('ref_axis',(1.,0.,0.));
#10510=DIRECTION('center_axis',(0.,1.,0.));
#10511=DIRECTION('ref_axis',(1.,0.,0.));
#10512=DIRECTION('center_axis',(0.,1.,0.));
#10513=DIRECTION('ref_axis',(1.,0.,0.));
#10514=DIRECTION('center_axis',(0.,1.,0.));
#10515=DIRECTION('ref_axis',(1.,0.,0.));
#10516=DIRECTION('',(0.,-1.,0.));
#10517=DIRECTION('center_axis',(0.,-1.,0.));
#10518=DIRECTION('ref_axis',(1.,0.,0.));
#10519=DIRECTION('center_axis',(0.,1.,0.));
#10520=DIRECTION('ref_axis',(1.,0.,0.));
#10521=DIRECTION('center_axis',(0.,1.,0.));
#10522=DIRECTION('ref_axis',(1.,0.,0.));
#10523=DIRECTION('center_axis',(0.,1.,0.));
#10524=DIRECTION('ref_axis',(1.,0.,0.));
#10525=DIRECTION('center_axis',(0.,1.,0.));
#10526=DIRECTION('ref_axis',(1.,0.,0.));
#10527=DIRECTION('center_axis',(0.,1.,0.));
#10528=DIRECTION('ref_axis',(1.,0.,0.));
#10529=DIRECTION('center_axis',(0.,1.,0.));
#10530=DIRECTION('ref_axis',(1.,0.,0.));
#10531=DIRECTION('center_axis',(0.,-1.,0.));
#10532=DIRECTION('ref_axis',(1.,0.,0.));
#10533=DIRECTION('center_axis',(0.,-1.,0.));
#10534=DIRECTION('ref_axis',(0.,0.,-1.));
#10535=DIRECTION('center_axis',(6.12323399573677E-17,0.,1.));
#10536=DIRECTION('ref_axis',(1.,0.,0.));
#10537=DIRECTION('center_axis',(0.,-1.,0.));
#10538=DIRECTION('ref_axis',(0.,0.,-1.));
#10539=DIRECTION('center_axis',(0.,1.,0.));
#10540=DIRECTION('ref_axis',(1.,0.,0.));
#10541=DIRECTION('center_axis',(0.,-1.,0.));
#10542=DIRECTION('ref_axis',(1.,0.,0.));
#10543=DIRECTION('center_axis',(0.,-1.,0.));
#10544=DIRECTION('ref_axis',(0.,0.,-1.));
#10545=DIRECTION('center_axis',(0.,0.,1.));
#10546=DIRECTION('ref_axis',(1.,0.,0.));
#10547=DIRECTION('center_axis',(0.,-1.,0.));
#10548=DIRECTION('ref_axis',(0.,0.,-1.));
#10549=DIRECTION('center_axis',(0.,1.,0.));
#10550=DIRECTION('ref_axis',(1.,0.,0.));
#10551=DIRECTION('center_axis',(0.,-1.,0.));
#10552=DIRECTION('ref_axis',(1.,0.,0.));
#10553=DIRECTION('center_axis',(0.,-1.,0.));
#10554=DIRECTION('ref_axis',(0.,0.,-1.));
#10555=DIRECTION('center_axis',(0.,0.,1.));
#10556=DIRECTION('ref_axis',(1.,0.,0.));
#10557=DIRECTION('center_axis',(0.,-1.,0.));
#10558=DIRECTION('ref_axis',(0.,0.,-1.));
#10559=DIRECTION('center_axis',(0.,1.,0.));
#10560=DIRECTION('ref_axis',(1.,0.,0.));
#10561=DIRECTION('center_axis',(0.,-1.,0.));
#10562=DIRECTION('ref_axis',(1.,0.,0.));
#10563=DIRECTION('center_axis',(0.,-1.,0.));
#10564=DIRECTION('ref_axis',(0.,0.,-1.));
#10565=DIRECTION('center_axis',(0.,0.,1.));
#10566=DIRECTION('ref_axis',(1.,0.,0.));
#10567=DIRECTION('center_axis',(0.,-1.,0.));
#10568=DIRECTION('ref_axis',(0.,0.,-1.));
#10569=DIRECTION('center_axis',(0.,1.,0.));
#10570=DIRECTION('ref_axis',(1.,0.,0.));
#10571=DIRECTION('center_axis',(0.,-1.,0.));
#10572=DIRECTION('ref_axis',(1.,0.,0.));
#10573=DIRECTION('center_axis',(0.,-1.,0.));
#10574=DIRECTION('ref_axis',(0.,0.,-1.));
#10575=DIRECTION('center_axis',(6.12323399573676E-17,0.,1.));
#10576=DIRECTION('ref_axis',(1.,0.,0.));
#10577=DIRECTION('center_axis',(0.,-1.,0.));
#10578=DIRECTION('ref_axis',(0.,0.,-1.));
#10579=DIRECTION('center_axis',(0.,1.,0.));
#10580=DIRECTION('ref_axis',(1.,0.,0.));
#10581=DIRECTION('center_axis',(0.,-1.,0.));
#10582=DIRECTION('ref_axis',(1.,0.,0.));
#10583=DIRECTION('center_axis',(0.,-1.,0.));
#10584=DIRECTION('ref_axis',(0.,0.,-1.));
#10585=DIRECTION('center_axis',(0.,0.,1.));
#10586=DIRECTION('ref_axis',(1.,0.,0.));
#10587=DIRECTION('center_axis',(0.,-1.,0.));
#10588=DIRECTION('ref_axis',(0.,0.,-1.));
#10589=DIRECTION('center_axis',(0.,1.,0.));
#10590=DIRECTION('ref_axis',(1.,0.,0.));
#10591=DIRECTION('center_axis',(0.,1.,0.));
#10592=DIRECTION('ref_axis',(1.,0.,0.));
#10593=DIRECTION('',(0.,1.,0.));
#10594=DIRECTION('center_axis',(0.,-1.,0.));
#10595=DIRECTION('ref_axis',(1.,0.,0.));
#10596=DIRECTION('center_axis',(0.,-1.,0.));
#10597=DIRECTION('ref_axis',(1.,0.,0.));
#10598=DIRECTION('center_axis',(0.,1.,0.));
#10599=DIRECTION('ref_axis',(1.,0.,0.));
#10600=DIRECTION('center_axis',(0.,-1.,0.));
#10601=DIRECTION('ref_axis',(0.,0.,-1.));
#10602=DIRECTION('center_axis',(0.,0.,1.));
#10603=DIRECTION('ref_axis',(1.,0.,0.));
#10604=DIRECTION('center_axis',(0.,-1.,0.));
#10605=DIRECTION('ref_axis',(0.,0.,-1.));
#10606=DIRECTION('center_axis',(0.,-1.,0.));
#10607=DIRECTION('ref_axis',(-1.,0.,0.));
#10608=DIRECTION('center_axis',(0.,1.,0.));
#10609=DIRECTION('ref_axis',(1.,0.,0.));
#13340=CARTESIAN_POINT('',(0.,0.,0.));
#13341=CARTESIAN_POINT('Origin',(0.707106781186547,0.,0.707106781186548));
#13342=CARTESIAN_POINT('',(0.504455939115715,-0.04763,0.841298510752802));
#13343=CARTESIAN_POINT('',(0.841298510752802,-0.04763,0.504455939115715));
#13344=CARTESIAN_POINT('Ctrl Pts',(0.504455939115715,-0.04763,0.841298510752802));
#13345=CARTESIAN_POINT('Ctrl Pts',(0.508899795931835,-0.0740444353928835,
0.838633903678357));
#13346=CARTESIAN_POINT('Ctrl Pts',(0.517157748491652,-0.0999305678883309,
0.833661031856294));
#13347=CARTESIAN_POINT('Ctrl Pts',(0.537715343527944,-0.142345102874864,
0.820511285096538));
#13348=CARTESIAN_POINT('Ctrl Pts',(0.548874290046456,-0.159766064500479,
0.813159949759));
#13349=CARTESIAN_POINT('Ctrl Pts',(0.573915184558107,-0.190326085855194,
0.795684265985089));
#13350=CARTESIAN_POINT('Ctrl Pts',(0.587792702767295,-0.203463743702801,
0.78555112003688));
#13351=CARTESIAN_POINT('Ctrl Pts',(0.615966552324775,-0.224161999508995,
0.763642258217233));
#13352=CARTESIAN_POINT('Ctrl Pts',(0.631684198665438,-0.232861760990032,
0.750785745543687));
#13353=CARTESIAN_POINT('Ctrl Pts',(0.663382628119203,-0.244251601209411,
0.722929908501543));
#13354=CARTESIAN_POINT('Ctrl Pts',(0.679352081686668,-0.246942143572133,
0.707917883896095));
#13355=CARTESIAN_POINT('Ctrl Pts',(0.707917883896095,-0.246942143572133,
0.679352081686668));
#13356=CARTESIAN_POINT('Ctrl Pts',(0.722929908501543,-0.244251601209411,
0.663382628119203));
#13357=CARTESIAN_POINT('Ctrl Pts',(0.750785745543687,-0.232861760990032,
0.631684198665439));
#13358=CARTESIAN_POINT('Ctrl Pts',(0.763642258217232,-0.224161999508995,
0.615966552324775));
#13359=CARTESIAN_POINT('Ctrl Pts',(0.78555112003688,-0.203463743702801,
0.587792702767295));
#13360=CARTESIAN_POINT('Ctrl Pts',(0.795684265985088,-0.190326085855194,
0.573915184558108));
#13361=CARTESIAN_POINT('Ctrl Pts',(0.813159949759,-0.15976606450048,0.548874290046456));
#13362=CARTESIAN_POINT('Ctrl Pts',(0.820511285096538,-0.142345102874864,
0.537715343527944));
#13363=CARTESIAN_POINT('Ctrl Pts',(0.833661031856294,-0.099930567888331,
0.517157748491653));
#13364=CARTESIAN_POINT('Ctrl Pts',(0.838633903678357,-0.0740444353928835,
0.508899795931835));
#13365=CARTESIAN_POINT('Ctrl Pts',(0.841298510752801,-0.0476299999999999,
0.504455939115715));
#13366=CARTESIAN_POINT('',(0.528110872004958,-0.04763,0.871530771444223));
#13367=CARTESIAN_POINT('Origin',(0.707106781186547,-0.04763,0.707106781186548));
#13368=CARTESIAN_POINT('',(0.871530771444223,-0.04763,0.528110872004959));
#13369=CARTESIAN_POINT('Ctrl Pts',(0.871530771444223,-0.0476300000000001,
0.528110872004958));
#13370=CARTESIAN_POINT('Ctrl Pts',(0.87014664509073,-0.0609922781173483,
0.530395067942936));
#13371=CARTESIAN_POINT('Ctrl Pts',(0.868149331745851,-0.0742967091364493,
0.533674141594226));
#13372=CARTESIAN_POINT('Ctrl Pts',(0.85981294420286,-0.115492077056649,
0.54708917182331));
#13373=CARTESIAN_POINT('Ctrl Pts',(0.850993704737257,-0.141695629206859,
0.560922177770136));
#13374=CARTESIAN_POINT('Ctrl Pts',(0.830754510485543,-0.181890537957859,
0.590422647829571));
#13375=CARTESIAN_POINT('Ctrl Pts',(0.816896541396381,-0.201072148666545,
0.609616703125488));
#13376=CARTESIAN_POINT('Ctrl Pts',(0.792310597819928,-0.223955109275652,
0.641117951819998));
#13377=CARTESIAN_POINT('Ctrl Pts',(0.779109323683612,-0.232742381310829,
0.657208095763053));
#13378=CARTESIAN_POINT('Ctrl Pts',(0.750552691816206,-0.244234834628584,
0.68964083160521));
#13379=CARTESIAN_POINT('Ctrl Pts',(0.735185187071673,-0.246942143572133,
0.705971972091755));
#13380=CARTESIAN_POINT('Ctrl Pts',(0.705971972091754,-0.246942143572133,
0.735185187071673));
#13381=CARTESIAN_POINT('Ctrl Pts',(0.689640831605209,-0.244234834628584,
0.750552691816206));
#13382=CARTESIAN_POINT('Ctrl Pts',(0.657208095763052,-0.232742381310829,
0.779109323683612));
#13383=CARTESIAN_POINT('Ctrl Pts',(0.641117951819998,-0.223955109275652,
0.792310597819928));
#13384=CARTESIAN_POINT('Ctrl Pts',(0.609616703125487,-0.201072148666545,
0.816896541396382));
#13385=CARTESIAN_POINT('Ctrl Pts',(0.590422647829571,-0.181890537957858,
0.830754510485544));
#13386=CARTESIAN_POINT('Ctrl Pts',(0.560922177770135,-0.141695629206858,
0.850993704737257));
#13387=CARTESIAN_POINT('Ctrl Pts',(0.547089171823309,-0.115492077056649,
0.859812944202861));
#13388=CARTESIAN_POINT('Ctrl Pts',(0.533674141594226,-0.0742967091364491,
0.868149331745852));
#13389=CARTESIAN_POINT('Ctrl Pts',(0.530395067942936,-0.0609922781173483,
0.870146645090731));
#13390=CARTESIAN_POINT('Ctrl Pts',(0.528110872004958,-0.0476300000000001,
0.871530771444223));
#13391=CARTESIAN_POINT('Origin',(0.707106781186547,-0.04763,0.707106781186548));
#13392=CARTESIAN_POINT('Origin',(0.,-0.166705,0.));
#13393=CARTESIAN_POINT('',(0.242834539687906,-0.04763,0.989696097314));
#13394=CARTESIAN_POINT('Origin',(0.,-0.04763,0.));
#13395=CARTESIAN_POINT('',(-0.242834539687907,-0.04763,0.989696097314));
#13396=CARTESIAN_POINT('Ctrl Pts',(0.242834539687906,-0.04763,0.989696097314));
#13397=CARTESIAN_POINT('Ctrl Pts',(0.24024064412003,-0.0609922781173483,
0.990332542620729));
#13398=CARTESIAN_POINT('Ctrl Pts',(0.236509675094874,-0.0742967091364492,
0.991238884025248));
#13399=CARTESIAN_POINT('Ctrl Pts',(0.221129100087819,-0.115492077056649,
0.994830026707808));
#13400=CARTESIAN_POINT('Ctrl Pts',(0.205111543747588,-0.141695629206859,
0.998375294985966));
#13401=CARTESIAN_POINT('Ctrl Pts',(0.169940289819232,-0.181890537957859,
1.00492400591205));
#13402=CARTESIAN_POINT('Ctrl Pts',(0.1465689792446,-0.201072148666545,1.00869718865384));
#13403=CARTESIAN_POINT('Ctrl Pts',(0.106909345252087,-0.223955109275652,
1.01358704779679));
#13404=CARTESIAN_POINT('Ctrl Pts',(0.0861971848975941,-0.232742381310829,
1.0156297872271));
#13405=CARTESIAN_POINT('Ctrl Pts',(0.0430711894098822,-0.244234834628584,
1.01837060663223));
#13406=CARTESIAN_POINT('Ctrl Pts',(0.0206568624125605,-0.246942143572133,
1.019052));
#13407=CARTESIAN_POINT('Ctrl Pts',(-0.0206568624125608,-0.246942143572133,
1.019052));
#13408=CARTESIAN_POINT('Ctrl Pts',(-0.0430711894098825,-0.244234834628584,
1.01837060663223));
#13409=CARTESIAN_POINT('Ctrl Pts',(-0.0861971848975943,-0.232742381310829,
1.0156297872271));
#13410=CARTESIAN_POINT('Ctrl Pts',(-0.106909345252088,-0.223955109275652,
1.01358704779679));
#13411=CARTESIAN_POINT('Ctrl Pts',(-0.1465689792446,-0.201072148666545,
1.00869718865384));
#13412=CARTESIAN_POINT('Ctrl Pts',(-0.169940289819232,-0.181890537957859,
1.00492400591205));
#13413=CARTESIAN_POINT('Ctrl Pts',(-0.205111543747588,-0.141695629206859,
0.998375294985966));
#13414=CARTESIAN_POINT('Ctrl Pts',(-0.221129100087819,-0.115492077056649,
0.994830026707808));
#13415=CARTESIAN_POINT('Ctrl Pts',(-0.236509675094875,-0.0742967091364493,
0.991238884025248));
#13416=CARTESIAN_POINT('Ctrl Pts',(-0.24024064412003,-0.0609922781173483,
0.990332542620729));
#13417=CARTESIAN_POINT('Ctrl Pts',(-0.242834539687907,-0.04763,0.989696097314));
#13418=CARTESIAN_POINT('',(-0.528110872004959,-0.04763,0.871530771444223));
#13419=CARTESIAN_POINT('Origin',(0.,-0.04763,0.));
#13420=CARTESIAN_POINT('',(-0.871530771444223,-0.04763,0.528110872004958));
#13421=CARTESIAN_POINT('Ctrl Pts',(-0.528110872004958,-0.0476300000000001,
0.871530771444223));
#13422=CARTESIAN_POINT('Ctrl Pts',(-0.530395067942936,-0.0609922781173484,
0.87014664509073));
#13423=CARTESIAN_POINT('Ctrl Pts',(-0.533674141594226,-0.0742967091364493,
0.868149331745851));
#13424=CARTESIAN_POINT('Ctrl Pts',(-0.54708917182331,-0.115492077056649,
0.85981294420286));
#13425=CARTESIAN_POINT('Ctrl Pts',(-0.560922177770136,-0.141695629206859,
0.850993704737257));
#13426=CARTESIAN_POINT('Ctrl Pts',(-0.590422647829571,-0.181890537957859,
0.830754510485543));
#13427=CARTESIAN_POINT('Ctrl Pts',(-0.609616703125488,-0.201072148666545,
0.816896541396381));
#13428=CARTESIAN_POINT('Ctrl Pts',(-0.641117951819998,-0.223955109275652,
0.792310597819928));
#13429=CARTESIAN_POINT('Ctrl Pts',(-0.657208095763053,-0.232742381310829,
0.779109323683611));
#13430=CARTESIAN_POINT('Ctrl Pts',(-0.68964083160521,-0.244234834628584,
0.750552691816205));
#13431=CARTESIAN_POINT('Ctrl Pts',(-0.705971972091755,-0.246942143572133,
0.735185187071673));
#13432=CARTESIAN_POINT('Ctrl Pts',(-0.735185187071673,-0.246942143572133,
0.705971972091754));
#13433=CARTESIAN_POINT('Ctrl Pts',(-0.750552691816206,-0.244234834628584,
0.689640831605209));
#13434=CARTESIAN_POINT('Ctrl Pts',(-0.779109323683612,-0.232742381310829,
0.657208095763052));
#13435=CARTESIAN_POINT('Ctrl Pts',(-0.792310597819928,-0.223955109275652,
0.641117951819998));
#13436=CARTESIAN_POINT('Ctrl Pts',(-0.816896541396382,-0.201072148666545,
0.609616703125487));
#13437=CARTESIAN_POINT('Ctrl Pts',(-0.830754510485544,-0.181890537957858,
0.590422647829571));
#13438=CARTESIAN_POINT('Ctrl Pts',(-0.850993704737257,-0.141695629206858,
0.560922177770135));
#13439=CARTESIAN_POINT('Ctrl Pts',(-0.859812944202861,-0.115492077056649,
0.547089171823309));
#13440=CARTESIAN_POINT('Ctrl Pts',(-0.868149331745852,-0.0742967091364491,
0.533674141594226));
#13441=CARTESIAN_POINT('Ctrl Pts',(-0.870146645090731,-0.0609922781173483,
0.530395067942936));
#13442=CARTESIAN_POINT('Ctrl Pts',(-0.871530771444223,-0.04763,0.528110872004958));
#13443=CARTESIAN_POINT('',(-0.989696097314,-0.04763,0.242834539687906));
#13444=CARTESIAN_POINT('Origin',(0.,-0.04763,0.));
#13445=CARTESIAN_POINT('',(-1.019052,-0.246942143572133,1.248489836334E-16));
#13446=CARTESIAN_POINT('Ctrl Pts',(-0.989696097314,-0.04763,0.242834539687906));
#13447=CARTESIAN_POINT('Ctrl Pts',(-0.990332542620729,-0.0609922781173483,
0.24024064412003));
#13448=CARTESIAN_POINT('Ctrl Pts',(-0.991238884025248,-0.0742967091364492,
0.236509675094874));
#13449=CARTESIAN_POINT('Ctrl Pts',(-0.994830026707808,-0.115492077056649,
0.221129100087819));
#13450=CARTESIAN_POINT('Ctrl Pts',(-0.998375294985966,-0.141695629206859,
0.205111543747588));
#13451=CARTESIAN_POINT('Ctrl Pts',(-1.00492400591205,-0.181890537957859,
0.169940289819232));
#13452=CARTESIAN_POINT('Ctrl Pts',(-1.00869718865384,-0.201072148666545,
0.1465689792446));
#13453=CARTESIAN_POINT('Ctrl Pts',(-1.01358704779679,-0.223955109275652,
0.106909345252088));
#13454=CARTESIAN_POINT('Ctrl Pts',(-1.0156297872271,-0.232742381310829,
0.0861971848975944));
#13455=CARTESIAN_POINT('Ctrl Pts',(-1.01837060663223,-0.244234834628584,
0.0430711894098825));
#13456=CARTESIAN_POINT('Ctrl Pts',(-1.019052,-0.246942143572133,0.0206568624125608));
#13457=CARTESIAN_POINT('Ctrl Pts',(-1.019052,-0.246942143572133,1.2490009027033E-16));
#13458=CARTESIAN_POINT('',(-1.019052,-0.28578,1.24797876996471E-16));
#13459=CARTESIAN_POINT('',(-1.019052,-0.166705,1.24797876996471E-16));
#13460=CARTESIAN_POINT('Origin',(0.,-0.28578,0.));
#13461=CARTESIAN_POINT('',(-0.989696097314,-0.04763,-0.242834539687906));
#13462=CARTESIAN_POINT('Ctrl Pts',(-1.019052,-0.246942143572133,1.2490009027033E-16));
#13463=CARTESIAN_POINT('Ctrl Pts',(-1.019052,-0.246942143572133,-0.0206568624125605));
#13464=CARTESIAN_POINT('Ctrl Pts',(-1.01837060663223,-0.244234834628584,
-0.0430711894098822));
#13465=CARTESIAN_POINT('Ctrl Pts',(-1.0156297872271,-0.232742381310829,
-0.0861971848975941));
#13466=CARTESIAN_POINT('Ctrl Pts',(-1.01358704779679,-0.223955109275652,
-0.106909345252087));
#13467=CARTESIAN_POINT('Ctrl Pts',(-1.00869718865384,-0.201072148666546,
-0.1465689792446));
#13468=CARTESIAN_POINT('Ctrl Pts',(-1.00492400591205,-0.181890537957859,
-0.169940289819232));
#13469=CARTESIAN_POINT('Ctrl Pts',(-0.998375294985966,-0.141695629206859,
-0.205111543747588));
#13470=CARTESIAN_POINT('Ctrl Pts',(-0.994830026707808,-0.11549207705665,
-0.221129100087819));
#13471=CARTESIAN_POINT('Ctrl Pts',(-0.991238884025248,-0.0742967091364495,
-0.236509675094874));
#13472=CARTESIAN_POINT('Ctrl Pts',(-0.990332542620729,-0.0609922781173484,
-0.24024064412003));
#13473=CARTESIAN_POINT('Ctrl Pts',(-0.989696097314,-0.0476300000000001,
-0.242834539687907));
#13474=CARTESIAN_POINT('',(-0.871530771444223,-0.04763,-0.528110872004958));
#13475=CARTESIAN_POINT('Origin',(0.,-0.04763,0.));
#13476=CARTESIAN_POINT('',(-0.528110872004958,-0.04763,-0.871530771444223));
#13477=CARTESIAN_POINT('Ctrl Pts',(-0.871530771444223,-0.0476300000000001,
-0.528110872004958));
#13478=CARTESIAN_POINT('Ctrl Pts',(-0.87014664509073,-0.0609922781173484,
-0.530395067942936));
#13479=CARTESIAN_POINT('Ctrl Pts',(-0.868149331745851,-0.0742967091364494,
-0.533674141594226));
#13480=CARTESIAN_POINT('Ctrl Pts',(-0.85981294420286,-0.115492077056649,
-0.54708917182331));
#13481=CARTESIAN_POINT('Ctrl Pts',(-0.850993704737257,-0.141695629206859,
-0.560922177770136));
#13482=CARTESIAN_POINT('Ctrl Pts',(-0.830754510485543,-0.181890537957859,
-0.590422647829571));
#13483=CARTESIAN_POINT('Ctrl Pts',(-0.816896541396381,-0.201072148666546,
-0.609616703125488));
#13484=CARTESIAN_POINT('Ctrl Pts',(-0.792310597819928,-0.223955109275652,
-0.641117951819999));
#13485=CARTESIAN_POINT('Ctrl Pts',(-0.779109323683611,-0.232742381310829,
-0.657208095763053));
#13486=CARTESIAN_POINT('Ctrl Pts',(-0.750552691816205,-0.244234834628584,
-0.68964083160521));
#13487=CARTESIAN_POINT('Ctrl Pts',(-0.735185187071673,-0.246942143572133,
-0.705971972091755));
#13488=CARTESIAN_POINT('Ctrl Pts',(-0.705971972091754,-0.246942143572133,
-0.735185187071673));
#13489=CARTESIAN_POINT('Ctrl Pts',(-0.68964083160521,-0.244234834628584,
-0.750552691816206));
#13490=CARTESIAN_POINT('Ctrl Pts',(-0.657208095763052,-0.232742381310829,
-0.779109323683612));
#13491=CARTESIAN_POINT('Ctrl Pts',(-0.641117951819998,-0.223955109275652,
-0.792310597819928));
#13492=CARTESIAN_POINT('Ctrl Pts',(-0.609616703125488,-0.201072148666545,
-0.816896541396381));
#13493=CARTESIAN_POINT('Ctrl Pts',(-0.590422647829571,-0.181890537957859,
-0.830754510485543));
#13494=CARTESIAN_POINT('Ctrl Pts',(-0.560922177770136,-0.141695629206859,
-0.850993704737257));
#13495=CARTESIAN_POINT('Ctrl Pts',(-0.54708917182331,-0.115492077056649,
-0.85981294420286));
#13496=CARTESIAN_POINT('Ctrl Pts',(-0.533674141594226,-0.0742967091364494,
-0.868149331745852));
#13497=CARTESIAN_POINT('Ctrl Pts',(-0.530395067942936,-0.0609922781173484,
-0.870146645090731));
#13498=CARTESIAN_POINT('Ctrl Pts',(-0.528110872004958,-0.0476300000000001,
-0.871530771444223));
#13499=CARTESIAN_POINT('',(-0.242834539687906,-0.04763,-0.989696097314));
#13500=CARTESIAN_POINT('Origin',(0.,-0.04763,0.));
#13501=CARTESIAN_POINT('',(0.242834539687906,-0.04763,-0.989696097314));
#13502=CARTESIAN_POINT('Ctrl Pts',(-0.242834539687907,-0.04763,-0.989696097314));
#13503=CARTESIAN_POINT('Ctrl Pts',(-0.24024064412003,-0.0609922781173483,
-0.990332542620729));
#13504=CARTESIAN_POINT('Ctrl Pts',(-0.236509675094874,-0.0742967091364493,
-0.991238884025248));
#13505=CARTESIAN_POINT('Ctrl Pts',(-0.221129100087819,-0.115492077056649,
-0.994830026707808));
#13506=CARTESIAN_POINT('Ctrl Pts',(-0.205111543747588,-0.141695629206859,
-0.998375294985966));
#13507=CARTESIAN_POINT('Ctrl Pts',(-0.169940289819232,-0.181890537957859,
-1.00492400591205));
#13508=CARTESIAN_POINT('Ctrl Pts',(-0.1465689792446,-0.201072148666545,
-1.00869718865384));
#13509=CARTESIAN_POINT('Ctrl Pts',(-0.106909345252087,-0.223955109275652,
-1.01358704779679));
#13510=CARTESIAN_POINT('Ctrl Pts',(-0.0861971848975942,-0.232742381310829,
-1.0156297872271));
#13511=CARTESIAN_POINT('Ctrl Pts',(-0.0430711894098823,-0.244234834628584,
-1.01837060663223));
#13512=CARTESIAN_POINT('Ctrl Pts',(-0.0206568624125606,-0.246942143572133,
-1.019052));
#13513=CARTESIAN_POINT('Ctrl Pts',(0.0206568624125607,-0.246942143572133,
-1.019052));
#13514=CARTESIAN_POINT('Ctrl Pts',(0.0430711894098824,-0.244234834628584,
-1.01837060663223));
#13515=CARTESIAN_POINT('Ctrl Pts',(0.0861971848975943,-0.232742381310829,
-1.0156297872271));
#13516=CARTESIAN_POINT('Ctrl Pts',(0.106909345252088,-0.223955109275652,
-1.01358704779679));
#13517=CARTESIAN_POINT('Ctrl Pts',(0.1465689792446,-0.201072148666545,-1.00869718865384));
#13518=CARTESIAN_POINT('Ctrl Pts',(0.169940289819232,-0.181890537957859,
-1.00492400591205));
#13519=CARTESIAN_POINT('Ctrl Pts',(0.205111543747588,-0.141695629206859,
-0.998375294985966));
#13520=CARTESIAN_POINT('Ctrl Pts',(0.221129100087819,-0.115492077056649,
-0.994830026707808));
#13521=CARTESIAN_POINT('Ctrl Pts',(0.236509675094874,-0.0742967091364493,
-0.991238884025248));
#13522=CARTESIAN_POINT('Ctrl Pts',(0.24024064412003,-0.0609922781173484,
-0.990332542620729));
#13523=CARTESIAN_POINT('Ctrl Pts',(0.242834539687907,-0.04763,-0.989696097314));
#13524=CARTESIAN_POINT('',(0.528110872004958,-0.04763,-0.871530771444223));
#13525=CARTESIAN_POINT('Origin',(0.,-0.04763,0.));
#13526=CARTESIAN_POINT('',(0.871530771444223,-0.04763,-0.528110872004958));
#13527=CARTESIAN_POINT('Ctrl Pts',(0.528110872004958,-0.0476300000000001,
-0.871530771444223));
#13528=CARTESIAN_POINT('Ctrl Pts',(0.530395067942936,-0.0609922781173484,
-0.870146645090731));
#13529=CARTESIAN_POINT('Ctrl Pts',(0.533674141594226,-0.0742967091364493,
-0.868149331745851));
#13530=CARTESIAN_POINT('Ctrl Pts',(0.54708917182331,-0.115492077056649,
-0.85981294420286));
#13531=CARTESIAN_POINT('Ctrl Pts',(0.560922177770136,-0.141695629206859,
-0.850993704737257));
#13532=CARTESIAN_POINT('Ctrl Pts',(0.590422647829571,-0.181890537957859,
-0.830754510485543));
#13533=CARTESIAN_POINT('Ctrl Pts',(0.609616703125488,-0.201072148666545,
-0.816896541396381));
#13534=CARTESIAN_POINT('Ctrl Pts',(0.641117951819998,-0.223955109275652,
-0.792310597819928));
#13535=CARTESIAN_POINT('Ctrl Pts',(0.657208095763053,-0.232742381310829,
-0.779109323683612));
#13536=CARTESIAN_POINT('Ctrl Pts',(0.68964083160521,-0.244234834628584,
-0.750552691816206));
#13537=CARTESIAN_POINT('Ctrl Pts',(0.705971972091755,-0.246942143572133,
-0.735185187071673));
#13538=CARTESIAN_POINT('Ctrl Pts',(0.735185187071673,-0.246942143572133,
-0.705971972091754));
#13539=CARTESIAN_POINT('Ctrl Pts',(0.750552691816206,-0.244234834628584,
-0.68964083160521));
#13540=CARTESIAN_POINT('Ctrl Pts',(0.779109323683612,-0.232742381310829,
-0.657208095763053));
#13541=CARTESIAN_POINT('Ctrl Pts',(0.792310597819928,-0.223955109275652,
-0.641117951819998));
#13542=CARTESIAN_POINT('Ctrl Pts',(0.816896541396381,-0.201072148666545,
-0.609616703125488));
#13543=CARTESIAN_POINT('Ctrl Pts',(0.830754510485543,-0.181890537957859,
-0.590422647829571));
#13544=CARTESIAN_POINT('Ctrl Pts',(0.850993704737257,-0.141695629206859,
-0.560922177770136));
#13545=CARTESIAN_POINT('Ctrl Pts',(0.85981294420286,-0.115492077056649,
-0.54708917182331));
#13546=CARTESIAN_POINT('Ctrl Pts',(0.868149331745851,-0.0742967091364493,
-0.533674141594226));
#13547=CARTESIAN_POINT('Ctrl Pts',(0.870146645090731,-0.0609922781173484,
-0.530395067942936));
#13548=CARTESIAN_POINT('Ctrl Pts',(0.871530771444223,-0.0476300000000001,
-0.528110872004958));
#13549=CARTESIAN_POINT('',(0.989696097314,-0.04763,-0.242834539687906));
#13550=CARTESIAN_POINT('Origin',(0.,-0.04763,0.));
#13551=CARTESIAN_POINT('',(0.989696097314,-0.04763,0.242834539687906));
#13552=CARTESIAN_POINT('Ctrl Pts',(0.989696097314,-0.04763,-0.242834539687907));
#13553=CARTESIAN_POINT('Ctrl Pts',(0.990332542620729,-0.0609922781173483,
-0.24024064412003));
#13554=CARTESIAN_POINT('Ctrl Pts',(0.991238884025248,-0.0742967091364493,
-0.236509675094874));
#13555=CARTESIAN_POINT('Ctrl Pts',(0.994830026707808,-0.115492077056649,
-0.221129100087819));
#13556=CARTESIAN_POINT('Ctrl Pts',(0.998375294985966,-0.141695629206859,
-0.205111543747588));
#13557=CARTESIAN_POINT('Ctrl Pts',(1.00492400591205,-0.181890537957859,
-0.169940289819232));
#13558=CARTESIAN_POINT('Ctrl Pts',(1.00869718865384,-0.201072148666545,
-0.1465689792446));
#13559=CARTESIAN_POINT('Ctrl Pts',(1.01358704779679,-0.223955109275652,
-0.106909345252087));
#13560=CARTESIAN_POINT('Ctrl Pts',(1.0156297872271,-0.232742381310829,-0.0861971848975942));
#13561=CARTESIAN_POINT('Ctrl Pts',(1.01837060663223,-0.244234834628584,
-0.0430711894098823));
#13562=CARTESIAN_POINT('Ctrl Pts',(1.019052,-0.246942143572133,-0.0206568624125607));
#13563=CARTESIAN_POINT('Ctrl Pts',(1.019052,-0.246942143572133,0.0206568624125607));
#13564=CARTESIAN_POINT('Ctrl Pts',(1.01837060663223,-0.244234834628584,
0.0430711894098823));
#13565=CARTESIAN_POINT('Ctrl Pts',(1.0156297872271,-0.232742381310829,0.0861971848975942));
#13566=CARTESIAN_POINT('Ctrl Pts',(1.01358704779679,-0.223955109275652,
0.106909345252087));
#13567=CARTESIAN_POINT('Ctrl Pts',(1.00869718865384,-0.201072148666545,
0.1465689792446));
#13568=CARTESIAN_POINT('Ctrl Pts',(1.00492400591205,-0.181890537957859,
0.169940289819232));
#13569=CARTESIAN_POINT('Ctrl Pts',(0.998375294985966,-0.141695629206859,
0.205111543747588));
#13570=CARTESIAN_POINT('Ctrl Pts',(0.994830026707808,-0.115492077056649,
0.221129100087819));
#13571=CARTESIAN_POINT('Ctrl Pts',(0.991238884025248,-0.0742967091364492,
0.236509675094874));
#13572=CARTESIAN_POINT('Ctrl Pts',(0.990332542620729,-0.0609922781173483,
0.24024064412003));
#13573=CARTESIAN_POINT('Ctrl Pts',(0.989696097314,-0.04763,0.242834539687907));
#13574=CARTESIAN_POINT('Origin',(0.,-0.04763,0.));
#13575=CARTESIAN_POINT('Origin',(0.,-0.04763,0.));
#13576=CARTESIAN_POINT('',(0.238183666596899,-0.04763,0.951592097314));
#13577=CARTESIAN_POINT('Origin',(0.,-0.04763,0.));
#13578=CARTESIAN_POINT('Origin',(-1.94289029309402E-16,-0.04763,1.));
#13579=CARTESIAN_POINT('Origin',(-1.94289029309402E-16,0.,1.));
#13580=CARTESIAN_POINT('',(-0.2381836665969,-0.04763,0.951592097314));
#13581=CARTESIAN_POINT('Ctrl Pts',(-0.238183666596899,-0.0476299999999999,
0.951592097314));
#13582=CARTESIAN_POINT('Ctrl Pts',(-0.233157223576062,-0.0740444353928835,
0.952850216871763));
#13583=CARTESIAN_POINT('Ctrl Pts',(-0.223801617934946,-0.0999305678883309,
0.955173119738174));
#13584=CARTESIAN_POINT('Ctrl Pts',(-0.199966927975188,-0.142345102874864,
0.960411259488514));
#13585=CARTESIAN_POINT('Ctrl Pts',(-0.1868781821531,-0.159766064500479,
0.963103647174702));
#13586=CARTESIAN_POINT('Ctrl Pts',(-0.15681442133453,-0.190326085855194,
0.968453058988463));
#13587=CARTESIAN_POINT('Ctrl Pts',(-0.139836317888043,-0.203463743702801,
0.971100730005489));
#13588=CARTESIAN_POINT('Ctrl Pts',(-0.104422493053067,-0.224161999508995,
0.975530745318961));
#13589=CARTESIAN_POINT('Ctrl Pts',(-0.0842175114474176,-0.232861760990032,
0.977553872336861));
#13590=CARTESIAN_POINT('Ctrl Pts',(-0.0421062857595701,-0.244251601209411,
0.980270995488453));
#13591=CARTESIAN_POINT('Ctrl Pts',(-0.0201990724523197,-0.246942143572133,
0.980948));
#13592=CARTESIAN_POINT('Ctrl Pts',(0.020199072452319,-0.246942143572133,
0.980948));
#13593=CARTESIAN_POINT('Ctrl Pts',(0.0421062857595694,-0.244251601209411,
0.980270995488454));
#13594=CARTESIAN_POINT('Ctrl Pts',(0.0842175114474169,-0.232861760990032,
0.977553872336861));
#13595=CARTESIAN_POINT('Ctrl Pts',(0.104422493053067,-0.224161999508995,
0.975530745318961));
#13596=CARTESIAN_POINT('Ctrl Pts',(0.139836317888042,-0.203463743702801,
0.971100730005489));
#13597=CARTESIAN_POINT('Ctrl Pts',(0.15681442133453,-0.190326085855194,
0.968453058988463));
#13598=CARTESIAN_POINT('Ctrl Pts',(0.1868781821531,-0.15976606450048,0.963103647174702));
#13599=CARTESIAN_POINT('Ctrl Pts',(0.199966927975188,-0.142345102874864,
0.960411259488514));
#13600=CARTESIAN_POINT('Ctrl Pts',(0.223801617934945,-0.0999305678883309,
0.955173119738174));
#13601=CARTESIAN_POINT('Ctrl Pts',(0.233157223576061,-0.0740444353928835,
0.952850216871763));
#13602=CARTESIAN_POINT('Ctrl Pts',(0.238183666596899,-0.0476299999999999,
0.951592097314));
#13603=CARTESIAN_POINT('Origin',(-1.94289029309402E-16,-0.04763,1.));
#13604=CARTESIAN_POINT('Origin',(0.,-0.04763,0.));
#13605=CARTESIAN_POINT('',(-0.504455939115715,-0.04763,0.841298510752802));
#13606=CARTESIAN_POINT('Origin',(0.,-0.04763,0.));
#13607=CARTESIAN_POINT('Origin',(-0.707106781186548,-0.04763,0.707106781186547));
#13608=CARTESIAN_POINT('Origin',(-0.707106781186548,0.,0.707106781186547));
#13609=CARTESIAN_POINT('',(-0.841298510752802,-0.04763,0.504455939115715));
#13610=CARTESIAN_POINT('Ctrl Pts',(-0.841298510752802,-0.04763,0.504455939115715));
#13611=CARTESIAN_POINT('Ctrl Pts',(-0.838633903678357,-0.0740444353928835,
0.508899795931835));
#13612=CARTESIAN_POINT('Ctrl Pts',(-0.833661031856294,-0.0999305678883309,
0.517157748491652));
#13613=CARTESIAN_POINT('Ctrl Pts',(-0.820511285096538,-0.142345102874864,
0.537715343527944));
#13614=CARTESIAN_POINT('Ctrl Pts',(-0.813159949759,-0.159766064500479,0.548874290046456));
#13615=CARTESIAN_POINT('Ctrl Pts',(-0.795684265985089,-0.190326085855194,
0.573915184558107));
#13616=CARTESIAN_POINT('Ctrl Pts',(-0.78555112003688,-0.203463743702801,
0.587792702767295));
#13617=CARTESIAN_POINT('Ctrl Pts',(-0.763642258217233,-0.224161999508995,
0.615966552324775));
#13618=CARTESIAN_POINT('Ctrl Pts',(-0.750785745543687,-0.232861760990032,
0.631684198665438));
#13619=CARTESIAN_POINT('Ctrl Pts',(-0.722929908501543,-0.244251601209411,
0.663382628119203));
#13620=CARTESIAN_POINT('Ctrl Pts',(-0.707917883896095,-0.246942143572133,
0.679352081686668));
#13621=CARTESIAN_POINT('Ctrl Pts',(-0.679352081686668,-0.246942143572133,
0.707917883896095));
#13622=CARTESIAN_POINT('Ctrl Pts',(-0.663382628119203,-0.244251601209411,
0.722929908501544));
#13623=CARTESIAN_POINT('Ctrl Pts',(-0.631684198665438,-0.232861760990031,
0.750785745543687));
#13624=CARTESIAN_POINT('Ctrl Pts',(-0.615966552324775,-0.224161999508995,
0.763642258217233));
#13625=CARTESIAN_POINT('Ctrl Pts',(-0.587792702767295,-0.203463743702801,
0.78555112003688));
#13626=CARTESIAN_POINT('Ctrl Pts',(-0.573915184558107,-0.190326085855194,
0.795684265985088));
#13627=CARTESIAN_POINT('Ctrl Pts',(-0.548874290046456,-0.159766064500479,
0.813159949759));
#13628=CARTESIAN_POINT('Ctrl Pts',(-0.537715343527944,-0.142345102874864,
0.820511285096538));
#13629=CARTESIAN_POINT('Ctrl Pts',(-0.517157748491652,-0.0999305678883309,
0.833661031856294));
#13630=CARTESIAN_POINT('Ctrl Pts',(-0.508899795931835,-0.0740444353928835,
0.838633903678357));
#13631=CARTESIAN_POINT('Ctrl Pts',(-0.504455939115716,-0.04763,0.841298510752801));
#13632=CARTESIAN_POINT('Origin',(-0.707106781186548,-0.04763,0.707106781186547));
#13633=CARTESIAN_POINT('Origin',(0.,-0.04763,0.));
#13634=CARTESIAN_POINT('',(-0.951592097314,-0.04763,0.238183666596899));
#13635=CARTESIAN_POINT('Origin',(0.,-0.04763,0.));
#13636=CARTESIAN_POINT('Origin',(-1.,-0.04763,-1.11022302462516E-16));
#13637=CARTESIAN_POINT('Origin',(-1.,0.,-1.11022302462516E-16));
#13638=CARTESIAN_POINT('',(-0.951592097314,-0.04763,-0.2381836665969));
#13639=CARTESIAN_POINT('',(-0.980948,-0.246942143572133,1.08514323328844E-18));
#13640=CARTESIAN_POINT('Ctrl Pts',(-0.951592097314,-0.04763,-0.238183666596899));
#13641=CARTESIAN_POINT('Ctrl Pts',(-0.952850216871763,-0.0740444353928835,
-0.233157223576062));
#13642=CARTESIAN_POINT('Ctrl Pts',(-0.955173119738174,-0.0999305678883309,
-0.223801617934946));
#13643=CARTESIAN_POINT('Ctrl Pts',(-0.960411259488514,-0.142345102874864,
-0.199966927975188));
#13644=CARTESIAN_POINT('Ctrl Pts',(-0.963103647174702,-0.159766064500479,
-0.1868781821531));
#13645=CARTESIAN_POINT('Ctrl Pts',(-0.968453058988463,-0.190326085855194,
-0.15681442133453));
#13646=CARTESIAN_POINT('Ctrl Pts',(-0.971100730005489,-0.203463743702801,
-0.139836317888043));
#13647=CARTESIAN_POINT('Ctrl Pts',(-0.975530745318961,-0.224161999508995,
-0.104422493053067));
#13648=CARTESIAN_POINT('Ctrl Pts',(-0.977553872336861,-0.232861760990032,
-0.0842175114474175));
#13649=CARTESIAN_POINT('Ctrl Pts',(-0.980270995488453,-0.244251601209411,
-0.0421062857595699));
#13650=CARTESIAN_POINT('Ctrl Pts',(-0.980948,-0.246942143572133,-0.0201990724523195));
#13651=CARTESIAN_POINT('Ctrl Pts',(-0.980948,-0.246942143572133,-1.17961196366423E-16));
#13652=CARTESIAN_POINT('Origin',(-1.,-0.04763,-1.11022302462516E-16));
#13653=CARTESIAN_POINT('Ctrl Pts',(-0.980948,-0.246942143572133,-1.17961196366423E-16));
#13654=CARTESIAN_POINT('Ctrl Pts',(-0.980948,-0.246942143572133,0.0201990724523192));
#13655=CARTESIAN_POINT('Ctrl Pts',(-0.980270995488453,-0.244251601209411,
0.0421062857595695));
#13656=CARTESIAN_POINT('Ctrl Pts',(-0.977553872336861,-0.232861760990032,
0.0842175114474169));
#13657=CARTESIAN_POINT('Ctrl Pts',(-0.975530745318961,-0.224161999508995,
0.104422493053066));
#13658=CARTESIAN_POINT('Ctrl Pts',(-0.971100730005489,-0.203463743702801,
0.139836317888042));
#13659=CARTESIAN_POINT('Ctrl Pts',(-0.968453058988463,-0.190326085855194,
0.15681442133453));
#13660=CARTESIAN_POINT('Ctrl Pts',(-0.963103647174702,-0.15976606450048,
0.1868781821531));
#13661=CARTESIAN_POINT('Ctrl Pts',(-0.960411259488514,-0.142345102874864,
0.199966927975188));
#13662=CARTESIAN_POINT('Ctrl Pts',(-0.955173119738174,-0.099930567888331,
0.223801617934945));
#13663=CARTESIAN_POINT('Ctrl Pts',(-0.952850216871763,-0.0740444353928835,
0.233157223576061));
#13664=CARTESIAN_POINT('Ctrl Pts',(-0.951592097314,-0.04763,0.238183666596899));
#13665=CARTESIAN_POINT('Origin',(0.,-0.04763,0.));
#13666=CARTESIAN_POINT('',(-0.841298510752802,-0.04763,-0.504455939115715));
#13667=CARTESIAN_POINT('Origin',(0.,-0.04763,0.));
#13668=CARTESIAN_POINT('Origin',(-0.707106781186547,-0.04763,-0.707106781186548));
#13669=CARTESIAN_POINT('Origin',(-0.707106781186547,0.,-0.707106781186548));
#13670=CARTESIAN_POINT('',(-0.504455939115715,-0.04763,-0.841298510752802));
#13671=CARTESIAN_POINT('Ctrl Pts',(-0.504455939115715,-0.04763,-0.841298510752802));
#13672=CARTESIAN_POINT('Ctrl Pts',(-0.508899795931835,-0.0740444353928835,
-0.838633903678357));
#13673=CARTESIAN_POINT('Ctrl Pts',(-0.517157748491652,-0.0999305678883309,
-0.833661031856294));
#13674=CARTESIAN_POINT('Ctrl Pts',(-0.537715343527944,-0.142345102874864,
-0.820511285096538));
#13675=CARTESIAN_POINT('Ctrl Pts',(-0.548874290046456,-0.159766064500479,
-0.813159949759));
#13676=CARTESIAN_POINT('Ctrl Pts',(-0.573915184558107,-0.190326085855194,
-0.795684265985089));
#13677=CARTESIAN_POINT('Ctrl Pts',(-0.587792702767295,-0.203463743702801,
-0.78555112003688));
#13678=CARTESIAN_POINT('Ctrl Pts',(-0.615966552324775,-0.224161999508995,
-0.763642258217233));
#13679=CARTESIAN_POINT('Ctrl Pts',(-0.631684198665438,-0.232861760990032,
-0.750785745543687));
#13680=CARTESIAN_POINT('Ctrl Pts',(-0.663382628119203,-0.244251601209411,
-0.722929908501543));
#13681=CARTESIAN_POINT('Ctrl Pts',(-0.679352081686668,-0.246942143572133,
-0.707917883896095));
#13682=CARTESIAN_POINT('Ctrl Pts',(-0.707917883896095,-0.246942143572133,
-0.679352081686668));
#13683=CARTESIAN_POINT('Ctrl Pts',(-0.722929908501543,-0.244251601209411,
-0.663382628119203));
#13684=CARTESIAN_POINT('Ctrl Pts',(-0.750785745543687,-0.232861760990032,
-0.631684198665439));
#13685=CARTESIAN_POINT('Ctrl Pts',(-0.763642258217232,-0.224161999508995,
-0.615966552324775));
#13686=CARTESIAN_POINT('Ctrl Pts',(-0.78555112003688,-0.203463743702801,
-0.587792702767295));
#13687=CARTESIAN_POINT('Ctrl Pts',(-0.795684265985088,-0.190326085855194,
-0.573915184558107));
#13688=CARTESIAN_POINT('Ctrl Pts',(-0.813159949759,-0.15976606450048,-0.548874290046456));
#13689=CARTESIAN_POINT('Ctrl Pts',(-0.820511285096538,-0.142345102874864,
-0.537715343527944));
#13690=CARTESIAN_POINT('Ctrl Pts',(-0.833661031856294,-0.0999305678883311,
-0.517157748491652));
#13691=CARTESIAN_POINT('Ctrl Pts',(-0.838633903678357,-0.0740444353928836,
-0.508899795931835));
#13692=CARTESIAN_POINT('Ctrl Pts',(-0.841298510752801,-0.04763,-0.504455939115715));
#13693=CARTESIAN_POINT('Origin',(-0.707106781186547,-0.04763,-0.707106781186548));
#13694=CARTESIAN_POINT('Origin',(0.,-0.04763,0.));
#13695=CARTESIAN_POINT('',(-0.238183666596899,-0.04763,-0.951592097314));
#13696=CARTESIAN_POINT('Origin',(0.,-0.04763,0.));
#13697=CARTESIAN_POINT('Origin',(5.55111512312578E-17,-0.04763,-1.));
#13698=CARTESIAN_POINT('Origin',(5.55111512312578E-17,0.,-1.));
#13699=CARTESIAN_POINT('',(0.238183666596899,-0.04763,-0.951592097314));
#13700=CARTESIAN_POINT('Ctrl Pts',(0.238183666596899,-0.04763,-0.951592097314));
#13701=CARTESIAN_POINT('Ctrl Pts',(0.233157223576062,-0.0740444353928835,
-0.952850216871763));
#13702=CARTESIAN_POINT('Ctrl Pts',(0.223801617934946,-0.099930567888331,
-0.955173119738174));
#13703=CARTESIAN_POINT('Ctrl Pts',(0.199966927975188,-0.142345102874864,
-0.960411259488514));
#13704=CARTESIAN_POINT('Ctrl Pts',(0.1868781821531,-0.15976606450048,-0.963103647174702));
#13705=CARTESIAN_POINT('Ctrl Pts',(0.15681442133453,-0.190326085855194,
-0.968453058988463));
#13706=CARTESIAN_POINT('Ctrl Pts',(0.139836317888042,-0.203463743702801,
-0.971100730005489));
#13707=CARTESIAN_POINT('Ctrl Pts',(0.104422493053067,-0.224161999508995,
-0.975530745318961));
#13708=CARTESIAN_POINT('Ctrl Pts',(0.0842175114474173,-0.232861760990032,
-0.977553872336861));
#13709=CARTESIAN_POINT('Ctrl Pts',(0.0421062857595698,-0.244251601209411,
-0.980270995488453));
#13710=CARTESIAN_POINT('Ctrl Pts',(0.0201990724523194,-0.246942143572133,
-0.980948));
#13711=CARTESIAN_POINT('Ctrl Pts',(-0.0201990724523193,-0.246942143572133,
-0.980948));
#13712=CARTESIAN_POINT('Ctrl Pts',(-0.0421062857595697,-0.244251601209411,
-0.980270995488453));
#13713=CARTESIAN_POINT('Ctrl Pts',(-0.0842175114474171,-0.232861760990032,
-0.977553872336861));
#13714=CARTESIAN_POINT('Ctrl Pts',(-0.104422493053067,-0.224161999508995,
-0.975530745318961));
#13715=CARTESIAN_POINT('Ctrl Pts',(-0.139836317888042,-0.203463743702801,
-0.971100730005489));
#13716=CARTESIAN_POINT('Ctrl Pts',(-0.15681442133453,-0.190326085855194,
-0.968453058988463));
#13717=CARTESIAN_POINT('Ctrl Pts',(-0.1868781821531,-0.15976606450048,-0.963103647174702));
#13718=CARTESIAN_POINT('Ctrl Pts',(-0.199966927975188,-0.142345102874864,
-0.960411259488514));
#13719=CARTESIAN_POINT('Ctrl Pts',(-0.223801617934945,-0.099930567888331,
-0.955173119738174));
#13720=CARTESIAN_POINT('Ctrl Pts',(-0.233157223576062,-0.0740444353928835,
-0.952850216871763));
#13721=CARTESIAN_POINT('Ctrl Pts',(-0.238183666596899,-0.0476299999999999,
-0.951592097314));
#13722=CARTESIAN_POINT('Origin',(5.55111512312578E-17,-0.04763,-1.));
#13723=CARTESIAN_POINT('Origin',(0.,-0.04763,0.));
#13724=CARTESIAN_POINT('',(0.504455939115715,-0.04763,-0.841298510752802));
#13725=CARTESIAN_POINT('Origin',(0.,-0.04763,0.));
#13726=CARTESIAN_POINT('Origin',(0.707106781186548,-0.04763,-0.707106781186547));
#13727=CARTESIAN_POINT('Origin',(0.707106781186548,0.,-0.707106781186547));
#13728=CARTESIAN_POINT('',(0.841298510752802,-0.04763,-0.504455939115715));
#13729=CARTESIAN_POINT('Ctrl Pts',(0.841298510752802,-0.04763,-0.504455939115715));
#13730=CARTESIAN_POINT('Ctrl Pts',(0.838633903678357,-0.0740444353928835,
-0.508899795931835));
#13731=CARTESIAN_POINT('Ctrl Pts',(0.833661031856294,-0.0999305678883309,
-0.517157748491652));
#13732=CARTESIAN_POINT('Ctrl Pts',(0.820511285096538,-0.142345102874864,
-0.537715343527944));
#13733=CARTESIAN_POINT('Ctrl Pts',(0.813159949759,-0.159766064500479,-0.548874290046456));
#13734=CARTESIAN_POINT('Ctrl Pts',(0.795684265985088,-0.190326085855194,
-0.573915184558107));
#13735=CARTESIAN_POINT('Ctrl Pts',(0.78555112003688,-0.203463743702801,
-0.587792702767295));
#13736=CARTESIAN_POINT('Ctrl Pts',(0.763642258217233,-0.224161999508995,
-0.615966552324775));
#13737=CARTESIAN_POINT('Ctrl Pts',(0.750785745543687,-0.232861760990032,
-0.631684198665438));
#13738=CARTESIAN_POINT('Ctrl Pts',(0.722929908501543,-0.244251601209411,
-0.663382628119203));
#13739=CARTESIAN_POINT('Ctrl Pts',(0.707917883896095,-0.246942143572133,
-0.679352081686668));
#13740=CARTESIAN_POINT('Ctrl Pts',(0.679352081686668,-0.246942143572133,
-0.707917883896095));
#13741=CARTESIAN_POINT('Ctrl Pts',(0.663382628119203,-0.244251601209411,
-0.722929908501543));
#13742=CARTESIAN_POINT('Ctrl Pts',(0.631684198665438,-0.232861760990032,
-0.750785745543687));
#13743=CARTESIAN_POINT('Ctrl Pts',(0.615966552324775,-0.224161999508995,
-0.763642258217232));
#13744=CARTESIAN_POINT('Ctrl Pts',(0.587792702767295,-0.203463743702801,
-0.78555112003688));
#13745=CARTESIAN_POINT('Ctrl Pts',(0.573915184558107,-0.190326085855194,
-0.795684265985088));
#13746=CARTESIAN_POINT('Ctrl Pts',(0.548874290046456,-0.159766064500479,
-0.813159949759));
#13747=CARTESIAN_POINT('Ctrl Pts',(0.537715343527944,-0.142345102874864,
-0.820511285096538));
#13748=CARTESIAN_POINT('Ctrl Pts',(0.517157748491652,-0.099930567888331,
-0.833661031856294));
#13749=CARTESIAN_POINT('Ctrl Pts',(0.508899795931835,-0.0740444353928835,
-0.838633903678357));
#13750=CARTESIAN_POINT('Ctrl Pts',(0.504455939115715,-0.04763,-0.841298510752801));
#13751=CARTESIAN_POINT('Origin',(0.707106781186548,-0.04763,-0.707106781186547));
#13752=CARTESIAN_POINT('Origin',(0.,-0.166705,0.));
#13753=CARTESIAN_POINT('',(-0.980948,-0.28578,1.20131482833E-16));
#13754=CARTESIAN_POINT('Origin',(0.,-0.28578,0.));
#13755=CARTESIAN_POINT('',(-0.980948,-0.166705,1.20131482833E-16));
#13756=CARTESIAN_POINT('',(0.951592097314,-0.04763,0.238183666596899));
#13757=CARTESIAN_POINT('Origin',(0.,-0.04763,0.));
#13758=CARTESIAN_POINT('',(0.951592097314,-0.04763,-0.238183666596899));
#13759=CARTESIAN_POINT('Ctrl Pts',(0.951592097314,-0.04763,0.238183666596899));
#13760=CARTESIAN_POINT('Ctrl Pts',(0.952850216871763,-0.0740444353928835,
0.233157223576062));
#13761=CARTESIAN_POINT('Ctrl Pts',(0.955173119738174,-0.099930567888331,
0.223801617934945));
#13762=CARTESIAN_POINT('Ctrl Pts',(0.960411259488514,-0.142345102874864,
0.199966927975188));
#13763=CARTESIAN_POINT('Ctrl Pts',(0.963103647174702,-0.15976606450048,
0.1868781821531));
#13764=CARTESIAN_POINT('Ctrl Pts',(0.968453058988463,-0.190326085855194,
0.15681442133453));
#13765=CARTESIAN_POINT('Ctrl Pts',(0.971100730005489,-0.203463743702801,
0.139836317888042));
#13766=CARTESIAN_POINT('Ctrl Pts',(0.975530745318961,-0.224161999508995,
0.104422493053067));
#13767=CARTESIAN_POINT('Ctrl Pts',(0.977553872336861,-0.232861760990032,
0.0842175114474172));
#13768=CARTESIAN_POINT('Ctrl Pts',(0.980270995488453,-0.244251601209411,
0.0421062857595697));
#13769=CARTESIAN_POINT('Ctrl Pts',(0.980948,-0.246942143572133,0.0201990724523194));
#13770=CARTESIAN_POINT('Ctrl Pts',(0.980948,-0.246942143572133,-0.0201990724523194));
#13771=CARTESIAN_POINT('Ctrl Pts',(0.980270995488453,-0.244251601209411,
-0.0421062857595697));
#13772=CARTESIAN_POINT('Ctrl Pts',(0.977553872336861,-0.232861760990032,
-0.0842175114474172));
#13773=CARTESIAN_POINT('Ctrl Pts',(0.975530745318961,-0.224161999508995,
-0.104422493053067));
#13774=CARTESIAN_POINT('Ctrl Pts',(0.971100730005489,-0.203463743702801,
-0.139836317888042));
#13775=CARTESIAN_POINT('Ctrl Pts',(0.968453058988463,-0.190326085855194,
-0.15681442133453));
#13776=CARTESIAN_POINT('Ctrl Pts',(0.963103647174702,-0.15976606450048,
-0.1868781821531));
#13777=CARTESIAN_POINT('Ctrl Pts',(0.960411259488514,-0.142345102874864,
-0.199966927975188));
#13778=CARTESIAN_POINT('Ctrl Pts',(0.955173119738174,-0.099930567888331,
-0.223801617934945));
#13779=CARTESIAN_POINT('Ctrl Pts',(0.952850216871763,-0.0740444353928835,
-0.233157223576062));
#13780=CARTESIAN_POINT('Ctrl Pts',(0.951592097314,-0.0476299999999999,-0.238183666596899));
#13781=CARTESIAN_POINT('Origin',(0.,-0.04763,0.));
#13782=CARTESIAN_POINT('Origin',(0.,-0.04763,0.));
#13783=CARTESIAN_POINT('Origin',(1.,-0.04763,0.));
#13784=CARTESIAN_POINT('Origin',(1.,0.,0.));
#13785=CARTESIAN_POINT('Origin',(1.,-0.04763,0.));
#13786=CARTESIAN_POINT('Origin',(0.,-0.28578,0.));
#13787=CARTESIAN_POINT('Origin',(0.,-0.04763,0.));
#14439=UNCERTAINTY_MEASURE_WITH_UNIT(LENGTH_MEASURE(0.001),#14513,
'DISTANCE_ACCURACY_VALUE',
'Maximum model space distance between geometric entities at asserted c
onnectivities');
#14455=UNCERTAINTY_MEASURE_WITH_UNIT(LENGTH_MEASURE(0.001),#14513,
'DISTANCE_ACCURACY_VALUE',
'Maximum model space distance between geometric entities at asserted c
onnectivities');
#14496=(
GEOMETRIC_REPRESENTATION_CONTEXT(3)
GLOBAL_UNCERTAINTY_ASSIGNED_CONTEXT((#14439))
GLOBAL_UNIT_ASSIGNED_CONTEXT((#14513,#14515,#14516))
REPRESENTATION_CONTEXT('','3D')
);
#14512=(
GEOMETRIC_REPRESENTATION_CONTEXT(3)
GLOBAL_UNCERTAINTY_ASSIGNED_CONTEXT((#14455))
GLOBAL_UNIT_ASSIGNED_CONTEXT((#14513,#14515,#14516))
REPRESENTATION_CONTEXT('','3D')
);
#14513=(
LENGTH_UNIT()
NAMED_UNIT(*)
SI_UNIT(.CENTI.,.METRE.)
);
#14515=(
NAMED_UNIT(*)
PLANE_ANGLE_UNIT()
SI_UNIT($,.RADIAN.)
);
#14516=(
NAMED_UNIT(*)
SI_UNIT($,.STERADIAN.)
SOLID_ANGLE_UNIT()
);
#14557=SHAPE_DEFINITION_REPRESENTATION(#14613,#14781);
#14613=PRODUCT_DEFINITION_SHAPE('',$,#14838);
#14781=SHAPE_REPRESENTATION('',(#8564),#14496);
#14797=PRODUCT_DEFINITION_CONTEXT('part definition',#14967,'design');
#14838=PRODUCT_DEFINITION('Cage','Cage',#14894,#14797);
#14894=PRODUCT_DEFINITION_FORMATION('',$,#15009);
#14967=APPLICATION_CONTEXT(
'Core Data for Automotive Mechanical Design Process');
#14968=PRODUCT_CONTEXT('part definition',#14967,'mechanical');
#15009=PRODUCT('Cage','Cage','Cage',(#14968));
#15081=COLOUR_RGB('Grey',0.48,0.52,0.57);
#15082=FILL_AREA_STYLE_COLOUR('',#15081);
#15083=FILL_AREA_STYLE('',(#15082));
#15084=SURFACE_STYLE_FILL_AREA(#15083);
#15085=SURFACE_SIDE_STYLE('',(#15084));
#15086=SURFACE_STYLE_USAGE(.BOTH.,#15085);
#15087=PRESENTATION_STYLE_ASSIGNMENT((#15086));
ENDSEC;
END-ISO-10303-21;
